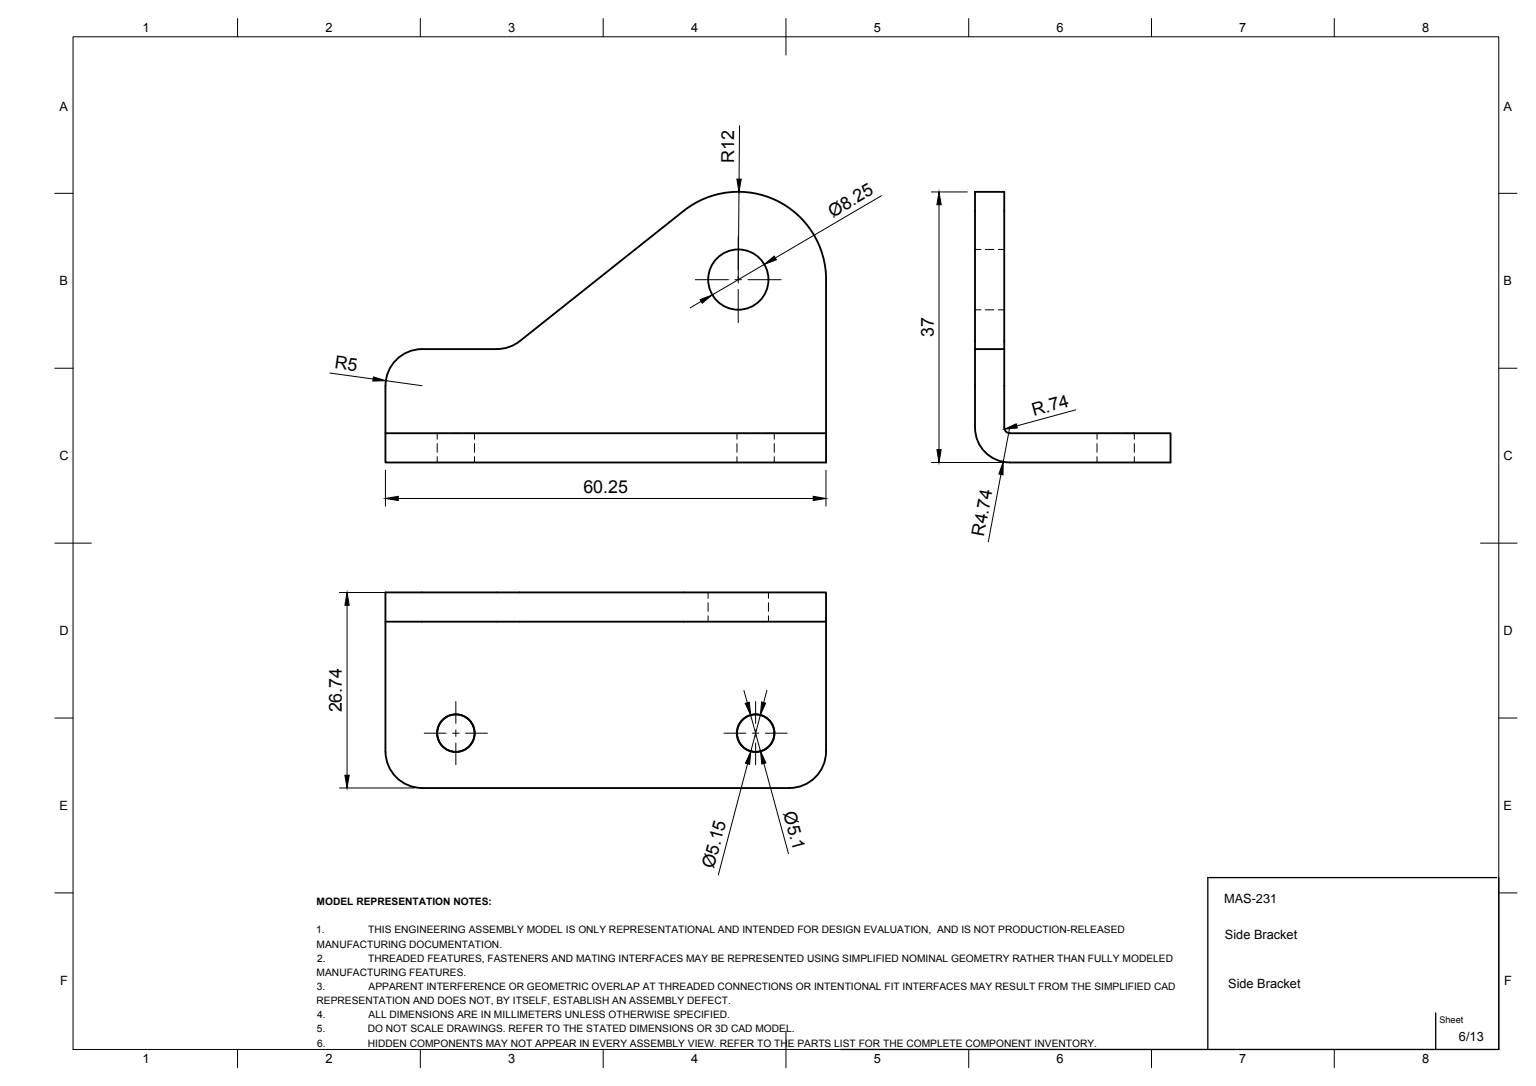
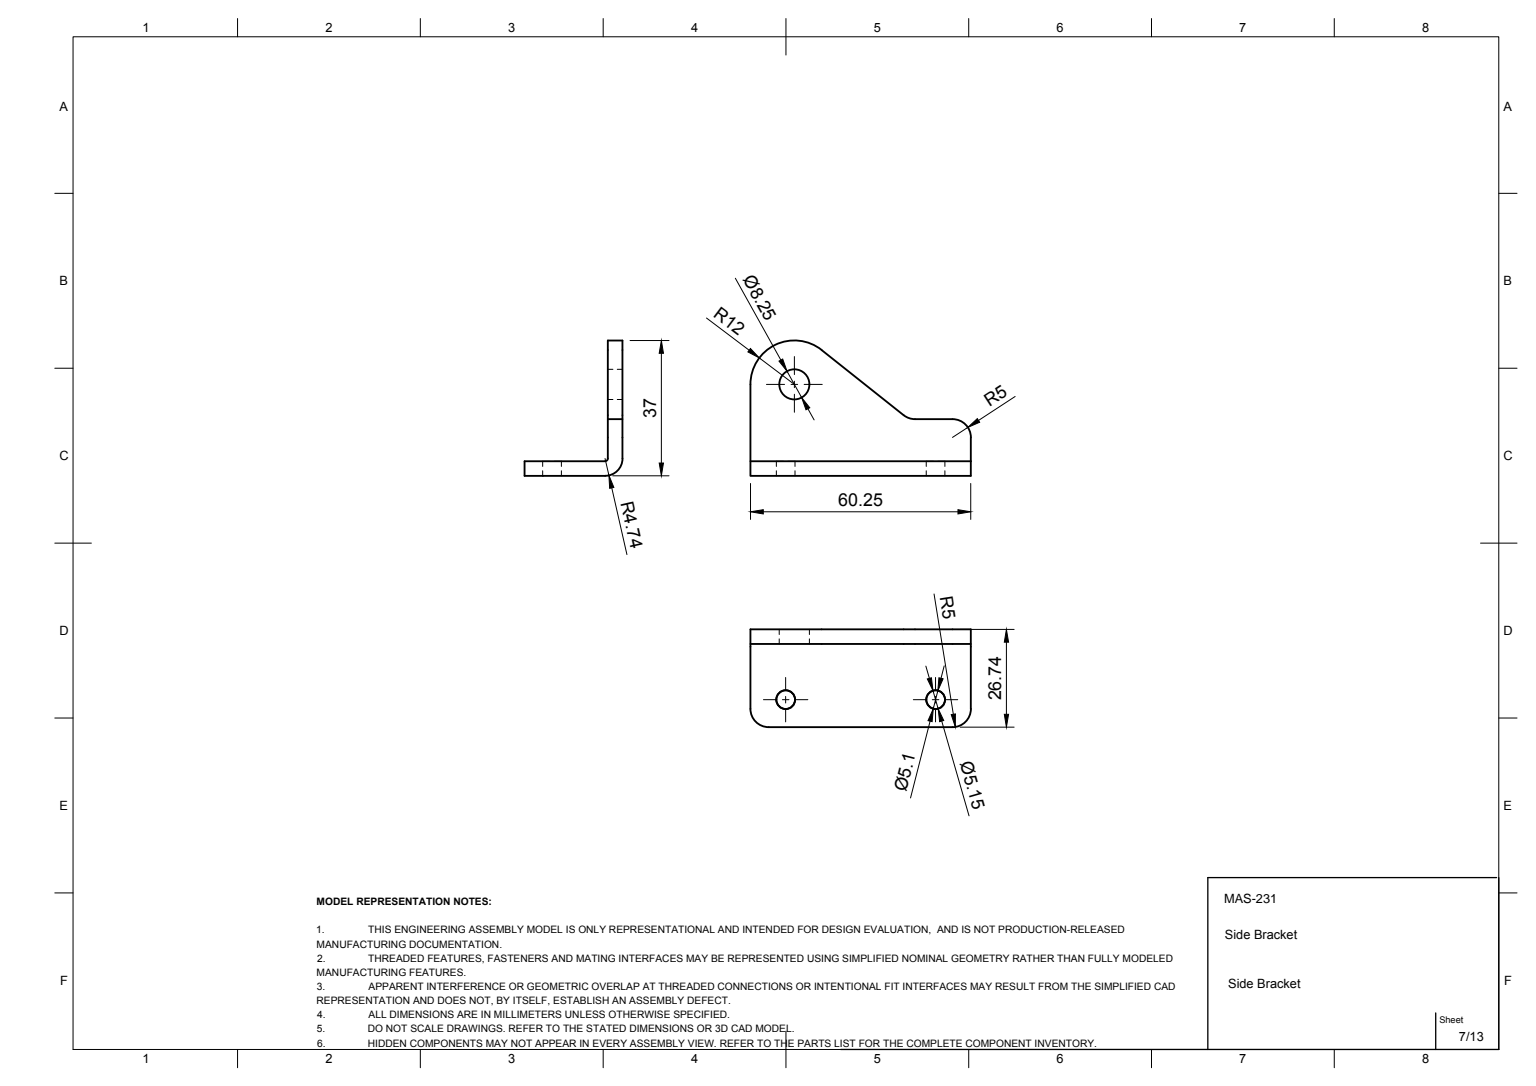
ISO-10303-21;
HEADER;
FILE_DESCRIPTION (('STEP AP214'),
    '1' );
FILE_NAME ( 'Side Bracket.step', '2026-10-04T02:08:54', ( '' ), ( '' ), 'STEP AP214', 'Unspecified', '' );
FILE_SCHEMA (( 'AUTOMOTIVE_DESIGN' ));
ENDSEC;
DATA;
#26=DIRECTION ( 'NONE',  ( 0.000000000000000000, 0.000000000000000000, -1.000000000000000000 ) ) ;
#60=VECTOR ( 'NONE', #5427, 39.37007874015748143 ) ;
#113=CARTESIAN_POINT ( 'NONE',  ( -0.6195511811023656223, 0.6102362204724407491, 1.186023622047243986 ) ) ;
#127=ORIENTED_EDGE ( 'NONE', *, *, #14895, .F. ) ;
#130=ADVANCED_FACE ( 'NONE', ( #15231 ), #18799, .T. ) ;
#143=DIRECTION ( 'NONE',  ( -0.000000000000000000, -0.000000000000000000, 1.000000000000000000 ) ) ;
#260=VECTOR ( 'NONE', #32837, 39.37007874015748143 ) ;
#351=DIRECTION ( 'NONE',  ( 0.000000000000000000, -0.6220299971367094782, 0.7829934116339071215 ) ) ;
#414=CARTESIAN_POINT ( 'NONE',  ( -0.4330708661417322913, 0.1574803149606299191, 1.186023622047243986 ) ) ;
#512=CARTESIAN_POINT ( 'NONE',  ( 0.1377952755905511861, -1.365923996832131609E-16, 0.9074803149606294195 ) ) ;
#523=ADVANCED_FACE ( 'NONE', ( #24362 ), #19359, .F. ) ;
#529=VERTEX_POINT ( 'NONE', #25560 ) ;
#593=CARTESIAN_POINT ( 'NONE',  ( -0.4620708661417322616, 0.6102362204724408601, 0.5854071585544579071 ) ) ;
#637=CARTESIAN_POINT ( 'NONE',  ( 0.1377952755905511861, 0.1574803149606299191, -0.7057086614173228023 ) ) ;
#705=DIRECTION ( 'NONE',  ( 0.000000000000000000, -1.000000000000000000, 0.000000000000000000 ) ) ;
#817=CIRCLE ( 'NONE', #6954, 0.1624015748031501782 ) ;
#870=DIRECTION ( 'NONE',  ( 1.000000000000000000, 0.000000000000000000, 0.000000000000000000 ) ) ;
#892=ORIENTED_EDGE ( 'NONE', *, *, #28438, .F. ) ;
#899=EDGE_CURVE ( 'NONE', #2549, #11279, #11446, .T. ) ;
#1038=CARTESIAN_POINT ( 'NONE',  ( 0.2362204724409448509, 0.000000000000000000, 0.9891732283464566011 ) ) ;
#1123=EDGE_CURVE ( 'NONE', #29994, #13605, #35169, .T. ) ;
#1148=VECTOR ( 'NONE', #44501, 39.37007874015748143 ) ;
#1243=AXIS2_PLACEMENT_3D ( 'NONE', #9459, #1527, #38204 ) ;
#1300=EDGE_CURVE ( 'NONE', #29883, #25085, #16051, .T. ) ;
#1356=ADVANCED_FACE ( 'NONE', ( #19336 ), #22697, .T. ) ;
#1362=LINE ( 'NONE', #9042, #21868 ) ;
#1430=DIRECTION ( 'NONE',  ( -0.000000000000000000, 1.000000000000000000, -0.000000000000000000 ) ) ;
#1435=AXIS2_PLACEMENT_3D ( 'NONE', #9624, #2406, #9388 ) ;
#1436=FACE_OUTER_BOUND ( 'NONE', #45627, .T. ) ;
#1527=DIRECTION ( 'NONE',  ( -1.000000000000000000, 0.000000000000000000, 0.000000000000000000 ) ) ;
#1544=CARTESIAN_POINT ( 'NONE',  ( -0.6195511811023656223, 1.354170115732555191, -0.4197102375732078561 ) ) ;
#1632=DIRECTION ( 'NONE',  ( 1.000000000000000000, 0.000000000000000000, 0.000000000000000000 ) ) ;
#1732=CARTESIAN_POINT ( 'NONE',  ( 0.2362204724409448509, 0.1574803149606299191, -1.186023622047243986 ) ) ;
#1811=CARTESIAN_POINT ( 'NONE',  ( -0.6195511811023656223, 0.6102362204724407491, 0.9891732283464566011 ) ) ;
#1826=FACE_OUTER_BOUND ( 'NONE', #11922, .T. ) ;
#1835=EDGE_LOOP ( 'NONE', ( #32627, #33041, #45588, #11414 ) ) ;
#1873=EDGE_CURVE ( 'NONE', #12155, #6854, #31803, .T. ) ;
#1938=VECTOR ( 'NONE', #4599, 39.37007874015748143 ) ;
#1969=DIRECTION ( 'NONE',  ( 0.000000000000000000, 0.000000000000000000, -1.000000000000000000 ) ) ;
#2028=DIRECTION ( 'NONE',  ( -1.000000000000000000, 0.000000000000000000, -0.000000000000000000 ) ) ;
#2073=ORIENTED_EDGE ( 'NONE', *, *, #24705, .F. ) ;
#2106=CARTESIAN_POINT ( 'NONE',  ( 0.1377952755905511861, 0.1574803149606299191, -0.8070866141732283561 ) ) ;
#2154=CYLINDRICAL_SURFACE ( 'NONE', #8738, 0.1003937007874010356 ) ;
#2261=ORIENTED_EDGE ( 'NONE', *, *, #17908, .T. ) ;
#2280=DIRECTION ( 'NONE',  ( 1.000000000000000000, 0.000000000000000000, 0.000000000000000000 ) ) ;
#2397=DIRECTION ( 'NONE',  ( 0.000000000000000000, -1.000000000000000000, 0.000000000000000000 ) ) ;
#2406=DIRECTION ( 'NONE',  ( 1.000000000000000000, 0.000000000000000000, 0.000000000000000000 ) ) ;
#2549=VERTEX_POINT ( 'NONE', #15817 ) ;
#2607=DIRECTION ( 'NONE',  ( 0.000000000000000000, 0.7071067811862592478, 0.7071067811868357866 ) ) ;
#2639=ADVANCED_FACE ( 'NONE', ( #36141 ), #42143, .F. ) ;
#2693=FACE_OUTER_BOUND ( 'NONE', #5912, .T. ) ;
#2716=CARTESIAN_POINT ( 'NONE',  ( 0.1377952755905511861, 0.1574803149606299191, 0.8070866141732283561 ) ) ;
#2735=AXIS2_PLACEMENT_3D ( 'NONE', #15622, #15860, #22308 ) ;
#2768=EDGE_LOOP ( 'NONE', ( #37512, #34957, #12199, #30879 ) ) ;
#2804=CARTESIAN_POINT ( 'NONE',  ( -0.6195511811023656223, 0.4133858267716533086, 0.9891732283464566011 ) ) ;
#2834=EDGE_LOOP ( 'NONE', ( #20225, #46223, #10055, #19298 ) ) ;
#2905=EDGE_CURVE ( 'NONE', #13605, #29883, #29414, .T. ) ;
#2998=DIRECTION ( 'NONE',  ( 1.000000000000000000, 0.000000000000000000, 0.000000000000000000 ) ) ;
#3054=DIRECTION ( 'NONE',  ( -0.000000000000000000, 1.000000000000000000, -0.000000000000000000 ) ) ;
#3076=EDGE_CURVE ( 'NONE', #35796, #18058, #15219, .T. ) ;
#3124=DIRECTION ( 'NONE',  ( -1.000000000000000000, -0.000000000000000000, -0.000000000000000000 ) ) ;
#3183=EDGE_CURVE ( 'NONE', #44249, #11279, #817, .T. ) ;
#3184=LINE ( 'NONE', #15175, #34310 ) ;
#3567=CARTESIAN_POINT ( 'NONE',  ( -0.4330708661417322913, 0.1574803149606299191, -1.186023622047243986 ) ) ;
#3624=ORIENTED_EDGE ( 'NONE', *, *, #6205, .F. ) ;
#3645=DIRECTION ( 'NONE',  ( 1.000000000000000000, -0.000000000000000000, -0.000000000000000000 ) ) ;
#3647=CARTESIAN_POINT ( 'NONE',  ( 0.1377952755905511861, 0.1574803149606299191, 0.8070866141732283561 ) ) ;
#3695=CARTESIAN_POINT ( 'NONE',  ( 0.2362204724409448509, 0.000000000000000000, -0.9891732283464566011 ) ) ;
#3759=DIRECTION ( 'NONE',  ( 0.000000000000000000, 0.000000000000000000, -1.000000000000000000 ) ) ;
#3854=ORIENTED_EDGE ( 'NONE', *, *, #16088, .T. ) ;
#3953=VERTEX_POINT ( 'NONE', #21496 ) ;
#4011=LINE ( 'NONE', #414, #45904 ) ;
#4021=AXIS2_PLACEMENT_3D ( 'NONE', #30055, #45315, #26672 ) ;
#4101=CARTESIAN_POINT ( 'NONE',  ( -0.6195511811023656223, 0.9842519685039375910, -0.7135826771653542844 ) ) ;
#4124=VERTEX_POINT ( 'NONE', #31468 ) ;
#4374=LINE ( 'NONE', #44870, #28589 ) ;
#4399=DIRECTION ( 'NONE',  ( 0.000000000000000000, -6.938893903907227392E-16, -1.000000000000000000 ) ) ;
#4455=AXIS2_PLACEMENT_3D ( 'NONE', #5889, #2280, #16908 ) ;
#4484=FACE_BOUND ( 'NONE', #14477, .T. ) ;
#4496=LINE ( 'NONE', #22739, #29482 ) ;
#4526=ADVANCED_FACE ( 'NONE', ( #12501 ), #2154, .F. ) ;
#4599=DIRECTION ( 'NONE',  ( 0.000000000000000000, 0.000000000000000000, -1.000000000000000000 ) ) ;
#4652=DIRECTION ( 'NONE',  ( 1.000000000000000000, -0.000000000000000000, -0.000000000000000000 ) ) ;
#4705=CARTESIAN_POINT ( 'NONE',  ( 0.1377952755905511861, 0.1564960629921262614, 0.8070866141732283561 ) ) ;
#4711=DIRECTION ( 'NONE',  ( 0.000000000000000000, -1.000000000000000000, 0.000000000000000000 ) ) ;
#4718=DIRECTION ( 'NONE',  ( -0.000000000000000000, 0.000000000000000000, 1.000000000000000000 ) ) ;
#4878=LINE ( 'NONE', #19504, #35583 ) ;
#4897=UNCERTAINTY_MEASURE_WITH_UNIT (LENGTH_MEASURE( 1.000000000000000082E-05 ), #37648, 'distance_accuracy_value', 'NONE') ;
#5034=AXIS2_PLACEMENT_3D ( 'NONE', #41786, #27710, #8985 ) ;
#5051=( LENGTH_UNIT ( ) NAMED_UNIT ( * ) SI_UNIT ( $, .METRE. ) ) ;
#5079=VERTEX_POINT ( 'NONE', #20073 ) ;
#5202=AXIS2_PLACEMENT_3D ( 'NONE', #8256, #4652, #37974 ) ;
#5208=CARTESIAN_POINT ( 'NONE',  ( 0.1377952755905512139, -1.365923996832131609E-16, -0.9074803149606294195 ) ) ;
#5223=CARTESIAN_POINT ( 'NONE',  ( -0.6195511811023656223, 0.000000000000000000, -1.186023622047243986 ) ) ;
#5224=CARTESIAN_POINT ( 'NONE',  ( -0.6195511811023656223, 0.4133858267716533086, 0.9891732283464566011 ) ) ;
#5284=PRESENTATION_STYLE_ASSIGNMENT (( #30489 ) ) ;
#5294=AXIS2_PLACEMENT_3D ( 'NONE', #3647, #25483, #21871 ) ;
#5427=DIRECTION ( 'NONE',  ( 1.000000000000000000, -0.000000000000000000, -0.000000000000000000 ) ) ;
#5572=CIRCLE ( 'NONE', #4021, 0.1624015748031501782 ) ;
#5598=DIRECTION ( 'NONE',  ( 0.000000000000000000, 0.000000000000000000, -1.000000000000000000 ) ) ;
#5659=CARTESIAN_POINT ( 'NONE',  ( 0.2362204724409448509, 0.1574803149606299191, -0.9891732283464566011 ) ) ;
#5702=CARTESIAN_POINT ( 'NONE',  ( 0.2362204724409448509, 0.000000000000000000, -0.9891732283464566011 ) ) ;
#5731=ORIENTED_EDGE ( 'NONE', *, *, #10353, .F. ) ;
#5743=DIRECTION ( 'NONE',  ( 8.659560562358463011E-17, 0.7071067811862592478, -0.7071067811868357866 ) ) ;
#5889=CARTESIAN_POINT ( 'NONE',  ( -0.6195511811023656223, 0.9842519685039370358, -0.7135826771653542844 ) ) ;
#5896=DIRECTION ( 'NONE',  ( -0.000000000000000000, 1.000000000000000000, -0.000000000000000000 ) ) ;
#5907=DIRECTION ( 'NONE',  ( 0.000000000000000000, 0.000000000000000000, 1.000000000000000000 ) ) ;
#5912=EDGE_LOOP ( 'NONE', ( #30515, #10422, #17857, #42784, #24375, #36154, #43440, #45182 ) ) ;
#5941=ORIENTED_EDGE ( 'NONE', *, *, #12634, .F. ) ;
#6011=EDGE_CURVE ( 'NONE', #43147, #15333, #1362, .T. ) ;
#6110=LINE ( 'NONE', #20734, #24316 ) ;
#6132=APPLICATION_CONTEXT ( 'automotive_design' ) ;
#6153=ORIENTED_EDGE ( 'NONE', *, *, #39860, .F. ) ;
#6205=EDGE_CURVE ( 'NONE', #22637, #43357, #7336, .T. ) ;
#6242=VECTOR ( 'NONE', #22207, 39.37007874015748143 ) ;
#6259=EDGE_CURVE ( 'NONE', #11279, #44249, #37154, .T. ) ;
#6289=DIRECTION ( 'NONE',  ( 0.000000000000000000, 1.000000000000000000, 0.000000000000000000 ) ) ;
#6308=LINE ( 'NONE', #24538, #22934 ) ;
#6350=ORIENTED_EDGE ( 'NONE', *, *, #35400, .T. ) ;
#6362=FACE_OUTER_BOUND ( 'NONE', #32085, .T. ) ;
#6381=EDGE_CURVE ( 'NONE', #3953, #17273, #33360, .T. ) ;
#6389=AXIS2_PLACEMENT_3D ( 'NONE', #21796, #15565, #30204 ) ;
#6414=CARTESIAN_POINT ( 'NONE',  ( 0.1377952755905512139, 0.1574803149606299191, 0.7066929133858274037 ) ) ;
#6442=ADVANCED_FACE ( 'NONE', ( #8507 ), #24088, .T. ) ;
#6446=EDGE_LOOP ( 'NONE', ( #33560, #24619, #11277, #8369 ) ) ;
#6451=DIRECTION ( 'NONE',  ( 0.000000000000000000, -0.000000000000000000, -1.000000000000000000 ) ) ;
#6518=CIRCLE ( 'NONE', #8063, 0.1013779527559055538 ) ;
#6533=DIRECTION ( 'NONE',  ( 0.000000000000000000, 1.000000000000000000, 0.000000000000000000 ) ) ;
#6658=FACE_OUTER_BOUND ( 'NONE', #42482, .T. ) ;
#6854=VERTEX_POINT ( 'NONE', #17889 ) ;
#6882=EDGE_LOOP ( 'NONE', ( #7362, #23755 ) ) ;
#6954=AXIS2_PLACEMENT_3D ( 'NONE', #43531, #25355, #3759 ) ;
#6982=CARTESIAN_POINT ( 'NONE',  ( 0.4330708661417322913, 0.1574803149606299191, -0.9891732283464566011 ) ) ;
#7140=CARTESIAN_POINT ( 'NONE',  ( 0.4330708661417322913, 0.000000000000000000, 0.9891732283464566011 ) ) ;
#7228=LENGTH_MEASURE_WITH_UNIT ( LENGTH_MEASURE( 0.02539999999999999897 ), #7455 ) ;
#7255=CARTESIAN_POINT ( 'NONE',  ( 0.2362204724409448509, 0.1574803149606299191, 1.186023622047243986 ) ) ;
#7294=FACE_OUTER_BOUND ( 'NONE', #24349, .T. ) ;
#7336=CIRCLE ( 'NONE', #16503, 0.1968503937007874405 ) ;
#7362=ORIENTED_EDGE ( 'NONE', *, *, #29891, .T. ) ;
#7455=( LENGTH_UNIT ( ) NAMED_UNIT ( * ) SI_UNIT ( $, .METRE. ) ) ;
#7562=DIRECTION ( 'NONE',  ( -1.000000000000000000, 0.000000000000000000, 0.000000000000000000 ) ) ;
#7622=EDGE_CURVE ( 'NONE', #42395, #24436, #30308, .T. ) ;
#7641=DIRECTION ( 'NONE',  ( 0.000000000000000000, 0.000000000000000000, 1.000000000000000000 ) ) ;
#7694=AXIS2_PLACEMENT_3D ( 'NONE', #31721, #9673, #17552 ) ;
#7700=CARTESIAN_POINT ( 'NONE',  ( 0.1377952755905511861, -1.365923996832131609E-16, 0.8070866141732283561 ) ) ;
#7771=DIRECTION ( 'NONE',  ( -1.000000000000000000, -0.000000000000000000, -0.000000000000000000 ) ) ;
#7800=CARTESIAN_POINT ( 'NONE',  ( 0.2362204724409448509, 0.1574803149606299191, 0.9891732283464566011 ) ) ;
#7922=ORIENTED_EDGE ( 'NONE', *, *, #14949, .F. ) ;
#8001=CARTESIAN_POINT ( 'NONE',  ( 0.1377952755905511861, 0.1564960629921262614, -0.8070866141732283561 ) ) ;
#8030=DIRECTION ( 'NONE',  ( 1.000000000000000000, -0.000000000000000000, -0.000000000000000000 ) ) ;
#8063=AXIS2_PLACEMENT_3D ( 'NONE', #8148, #705, #15363 ) ;
#8148=CARTESIAN_POINT ( 'NONE',  ( 0.1377952755905511861, 0.1574803149606299191, -0.8070866141732283561 ) ) ;
#8167=DIRECTION ( 'NONE',  ( 0.000000000000000000, 0.000000000000000000, 1.000000000000000000 ) ) ;
#8193=ORIENTED_EDGE ( 'NONE', *, *, #31586, .T. ) ;
#8253=DIRECTION ( 'NONE',  ( -0.000000000000000000, 0.7829934116339072325, 0.6220299971367095893 ) ) ;
#8256=CARTESIAN_POINT ( 'NONE',  ( -0.4620708661417322616, 0.9842519685039375910, -0.7135826771653542844 ) ) ;
#8369=ORIENTED_EDGE ( 'NONE', *, *, #27138, .F. ) ;
#8417=ORIENTED_EDGE ( 'NONE', *, *, #28893, .F. ) ;
#8475=CIRCLE ( 'NONE', #33010, 0.1864803149606299171 ) ;
#8507=FACE_OUTER_BOUND ( 'NONE', #29134, .T. ) ;
#8581=CIRCLE ( 'NONE', #24674, 0.1624015748031501782 ) ;
#8585=CARTESIAN_POINT ( 'NONE',  ( -0.4330708661417356775, 0.1864803149606299171, 1.186023622047243986 ) ) ;
#8653=EDGE_CURVE ( 'NONE', #43692, #16170, #6518, .T. ) ;
#8709=ORIENTED_EDGE ( 'NONE', *, *, #11424, .F. ) ;
#8738=AXIS2_PLACEMENT_3D ( 'NONE', #44808, #1430, #41675 ) ;
#8756=EDGE_CURVE ( 'NONE', #35268, #16170, #24432, .T. ) ;
#8833=LINE ( 'NONE', #5223, #25116 ) ;
#8834=FACE_OUTER_BOUND ( 'NONE', #6446, .T. ) ;
#8855=ORIENTED_EDGE ( 'NONE', *, *, #40556, .F. ) ;
#8985=DIRECTION ( 'NONE',  ( 0.000000000000000000, 0.000000000000000000, 1.000000000000000000 ) ) ;
#9042=CARTESIAN_POINT ( 'NONE',  ( 0.1377952755905512139, 0.1574803149606299191, -0.9074803149606294195 ) ) ;
#9307=EDGE_CURVE ( 'NONE', #12155, #29873, #41016, .T. ) ;
#9322=ORIENTED_EDGE ( 'NONE', *, *, #2905, .F. ) ;
#9377=FACE_BOUND ( 'NONE', #18186, .T. ) ;
#9388=DIRECTION ( 'NONE',  ( 0.000000000000000000, 0.000000000000000000, -1.000000000000000000 ) ) ;
#9459=CARTESIAN_POINT ( 'NONE',  ( 0.4330708661417322913, 0.000000000000000000, 0.000000000000000000 ) ) ;
#9573=CARTESIAN_POINT ( 'NONE',  ( -0.4620708661417322616, 0.6529540528279709211, 0.4629603087243971959 ) ) ;
#9624=CARTESIAN_POINT ( 'NONE',  ( -0.6195511811023656223, 0.8070866141732282451, 0.5854071585544579071 ) ) ;
#9633=ORIENTED_EDGE ( 'NONE', *, *, #47238, .F. ) ;
#9643=ORIENTED_EDGE ( 'NONE', *, *, #26702, .F. ) ;
#9673=DIRECTION ( 'NONE',  ( 1.000000000000000000, 0.000000000000000000, 0.000000000000000000 ) ) ;
#9681=DIRECTION ( 'NONE',  ( 1.000000000000000000, 0.000000000000000000, 0.000000000000000000 ) ) ;
#9700=ORIENTED_EDGE ( 'NONE', *, *, #20244, .T. ) ;
#9746=DIRECTION ( 'NONE',  ( 1.000000000000000000, 0.000000000000000000, 0.000000000000000000 ) ) ;
#9869=EDGE_LOOP ( 'NONE', ( #5731, #22652, #45000, #25793 ) ) ;
#9905=LINE ( 'NONE', #39113, #37079 ) ;
#9974=DIRECTION ( 'NONE',  ( 0.000000000000000000, 0.000000000000000000, -1.000000000000000000 ) ) ;
#9992=ORIENTED_EDGE ( 'NONE', *, *, #14895, .T. ) ;
#10018=DIRECTION ( 'NONE',  ( 0.000000000000000000, 0.000000000000000000, -1.000000000000000000 ) ) ;
#10032=AXIS2_PLACEMENT_3D ( 'NONE', #5224, #19854, #27798 ) ;
#10055=ORIENTED_EDGE ( 'NONE', *, *, #3183, .T. ) ;
#10270=DIRECTION ( 'NONE',  ( -0.000000000000000000, 1.000000000000000000, -0.000000000000000000 ) ) ;
#10274=LINE ( 'NONE', #7140, #25258 ) ;
#10313=DIRECTION ( 'NONE',  ( 0.000000000000000000, 0.000000000000000000, -1.000000000000000000 ) ) ;
#10353=EDGE_CURVE ( 'NONE', #3953, #40227, #17444, .T. ) ;
#10422=ORIENTED_EDGE ( 'NONE', *, *, #22465, .T. ) ;
#10470=ORIENTED_EDGE ( 'NONE', *, *, #20770, .T. ) ;
#10479=ORIENTED_EDGE ( 'NONE', *, *, #6205, .T. ) ;
#10502=CARTESIAN_POINT ( 'NONE',  ( -0.6195511811023656223, 0.1864803149606299171, -1.186023622047243986 ) ) ;
#10505=DIRECTION ( 'NONE',  ( -1.000000000000000000, -0.000000000000000000, -0.000000000000000000 ) ) ;
#10513=CYLINDRICAL_SURFACE ( 'NONE', #36435, 0.1003937007874010356 ) ;
#10628=EDGE_CURVE ( 'NONE', #13680, #25085, #6110, .T. ) ;
#10784=ORIENTED_EDGE ( 'NONE', *, *, #6381, .T. ) ;
#10835=DIRECTION ( 'NONE',  ( 1.000000000000000000, 0.000000000000000000, 0.000000000000000000 ) ) ;
#10911=DIRECTION ( 'NONE',  ( 0.000000000000000000, 0.000000000000000000, -1.000000000000000000 ) ) ;
#11221=ADVANCED_FACE ( 'NONE', ( #41058 ), #19033, .F. ) ;
#11265=FACE_BOUND ( 'NONE', #46562, .T. ) ;
#11277=ORIENTED_EDGE ( 'NONE', *, *, #22465, .F. ) ;
#11279=VERTEX_POINT ( 'NONE', #20461 ) ;
#11414=ORIENTED_EDGE ( 'NONE', *, *, #6259, .T. ) ;
#11424=EDGE_CURVE ( 'NONE', #25085, #29994, #3184, .T. ) ;
#11446=LINE ( 'NONE', #37295, #19059 ) ;
#11453=DIRECTION ( 'NONE',  ( 0.000000000000000000, 0.000000000000000000, -1.000000000000000000 ) ) ;
#11510=ORIENTED_EDGE ( 'NONE', *, *, #25210, .F. ) ;
#11597=DIRECTION ( 'NONE',  ( 0.000000000000000000, 0.7071067811862592478, 0.7071067811868357866 ) ) ;
#11712=DIRECTION ( 'NONE',  ( 1.000000000000000000, 0.000000000000000000, 0.000000000000000000 ) ) ;
#11733=CARTESIAN_POINT ( 'NONE',  ( -0.4620708661417322616, 0.9842519685039375910, -0.7135826771653542844 ) ) ;
#11743=ORIENTED_EDGE ( 'NONE', *, *, #20979, .F. ) ;
#11787=( NAMED_UNIT ( * ) SI_UNIT ( $, .STERADIAN. ) SOLID_ANGLE_UNIT ( ) ) ;
#11794=( NAMED_UNIT ( * ) PLANE_ANGLE_UNIT ( ) SI_UNIT ( $, .RADIAN. ) ) ;
#11827=EDGE_LOOP ( 'NONE', ( #32231, #43129, #27996, #7922 ) ) ;
#11859=CARTESIAN_POINT ( 'NONE',  ( -0.6195511811023656223, 0.6102362204724408601, 0.5854071585544579071 ) ) ;
#11877=ORIENTED_EDGE ( 'NONE', *, *, #17908, .F. ) ;
#11922=EDGE_LOOP ( 'NONE', ( #18416, #10479, #15708, #9700, #46879, #16747 ) ) ;
#11944=PRODUCT_DEFINITION ( 'UNKNOWN', '', #26300, #18289 ) ;
#12098=CIRCLE ( 'NONE', #24332, 0.1003937007874010356 ) ;
#12155=VERTEX_POINT ( 'NONE', #16762 ) ;
#12190=CIRCLE ( 'NONE', #39696, 0.1968503937007874405 ) ;
#12199=ORIENTED_EDGE ( 'NONE', *, *, #45641, .F. ) ;
#12200=CYLINDRICAL_SURFACE ( 'NONE', #33811, 0.1864803149606299171 ) ;
#12253=VERTEX_POINT ( 'NONE', #38327 ) ;
#12448=CIRCLE ( 'NONE', #32360, 0.1864803149606299448 ) ;
#12501=FACE_OUTER_BOUND ( 'NONE', #9869, .T. ) ;
#12510=SURFACE_SIDE_STYLE ('',( #34082 ) ) ;
#12551=DIRECTION ( 'NONE',  ( -1.000000000000000000, 0.000000000000000000, 0.000000000000000000 ) ) ;
#12558=CARTESIAN_POINT ( 'NONE',  ( 0.1377952755905512139, 0.1574803149606299191, -0.9084645669291339098 ) ) ;
#12600=EDGE_LOOP ( 'NONE', ( #35339, #13655, #8417, #36103 ) ) ;
#12634=EDGE_CURVE ( 'NONE', #15333, #43692, #15848, .T. ) ;
#12815=CARTESIAN_POINT ( 'NONE',  ( 0.1377952755905511861, 0.1564960629921262614, 0.8070866141732283561 ) ) ;
#12911=DIRECTION ( 'NONE',  ( 0.000000000000000000, 1.000000000000000000, 0.000000000000000000 ) ) ;
#12994=CARTESIAN_POINT ( 'NONE',  ( 0.4330708661417322913, 0.1574803149606299191, 1.186023622047243986 ) ) ;
#13111=CARTESIAN_POINT ( 'NONE',  ( 0.4330708661417322913, 0.000000000000000000, 0.9891732283464564901 ) ) ;
#13161=DIRECTION ( 'NONE',  ( 0.000000000000000000, 0.000000000000000000, -1.000000000000000000 ) ) ;
#13215=COLOUR_RGB ( '', 0.66274510, 0.83137255, 0.94901961) ;
#13306=ORIENTED_EDGE ( 'NONE', *, *, #44495, .F. ) ;
#13461=CARTESIAN_POINT ( 'NONE',  ( 0.1377952755905512139, 0.1564960629921262614, -0.9074803149606294195 ) ) ;
#13564=CARTESIAN_POINT ( 'NONE',  ( -0.6195511811023656223, 0.000000000000000000, 1.186023622047243986 ) ) ;
#13605=VERTEX_POINT ( 'NONE', #593 ) ;
#13645=ADVANCED_FACE ( 'NONE', ( #17881 ), #29200, .F. ) ;
#13655=ORIENTED_EDGE ( 'NONE', *, *, #33256, .T. ) ;
#13680=VERTEX_POINT ( 'NONE', #1544 ) ;
#13729=CARTESIAN_POINT ( 'NONE',  ( -0.4620708661417322616, 0.9842519685039370358, -1.186023622047243986 ) ) ;
#13748=ORIENTED_EDGE ( 'NONE', *, *, #33855, .F. ) ;
#13760=ORIENTED_EDGE ( 'NONE', *, *, #24727, .F. ) ;
#13795=EDGE_LOOP ( 'NONE', ( #27097, #46225, #17036, #10470 ) ) ;
#13889=CARTESIAN_POINT ( 'NONE',  ( -0.4620708661417322616, 0.1864803149606299448, -0.7135826771653542844 ) ) ;
#13892=AXIS2_PLACEMENT_3D ( 'NONE', #21219, #21709, #43737 ) ;
#13933=ORIENTED_EDGE ( 'NONE', *, *, #16088, .F. ) ;
#13934=AXIS2_PLACEMENT_3D ( 'NONE', #2804, #10505, #10018 ) ;
#13957=DIRECTION ( 'NONE',  ( 8.659560562358463011E-17, 0.7071067811862592478, -0.7071067811868357866 ) ) ;
#14001=FACE_OUTER_BOUND ( 'NONE', #19415, .T. ) ;
#14164=ORIENTED_EDGE ( 'NONE', *, *, #30136, .F. ) ;
#14214=PLANE ( 'NONE',  #7694 ) ;
#14338=CARTESIAN_POINT ( 'NONE',  ( 0.1377952755905511861, 0.1564960629921262614, 0.8070866141732283561 ) ) ;
#14343=CYLINDRICAL_SURFACE ( 'NONE', #40544, 0.1003937007874010356 ) ;
#14419=AXIS2_PLACEMENT_3D ( 'NONE', #29743, #40457, #7641 ) ;
#14477=EDGE_LOOP ( 'NONE', ( #29063, #6350 ) ) ;
#14589=CARTESIAN_POINT ( 'NONE',  ( 0.4330708661417322913, 0.000000000000000000, -0.9891732283464566011 ) ) ;
#14590=PRODUCT ( 'Side Bracket', 'Side Bracket', '', ( #16610 ) ) ;
#14602=PLANE ( 'NONE',  #6389 ) ;
#14607=CARTESIAN_POINT ( 'NONE',  ( -0.4620708661417322616, 0.1864803149606299448, 1.186023622047243986 ) ) ;
#14748=CARTESIAN_POINT ( 'NONE',  ( -0.4620708661417322616, 0.8070866141732282451, 0.5854071585544579071 ) ) ;
#14752=DIRECTION ( 'NONE',  ( 1.000000000000000000, 0.000000000000000000, 0.000000000000000000 ) ) ;
#14895=EDGE_CURVE ( 'NONE', #46399, #37690, #6308, .T. ) ;
#14949=EDGE_CURVE ( 'NONE', #46224, #24436, #18354, .T. ) ;
#15079=VERTEX_POINT ( 'NONE', #30062 ) ;
#15167=ORIENTED_EDGE ( 'NONE', *, *, #46577, .T. ) ;
#15175=CARTESIAN_POINT ( 'NONE',  ( -0.4620708661417322616, 0.6529540528279709211, 0.4629603087243968074 ) ) ;
#15219=LINE ( 'NONE', #29868, #42913 ) ;
#15231=FACE_OUTER_BOUND ( 'NONE', #2768, .T. ) ;
#15258=AXIS2_PLACEMENT_3D ( 'NONE', #44021, #870, #11453 ) ;
#15298=CARTESIAN_POINT ( 'NONE',  ( -0.4330708661417322913, 0.1864803149606299448, 1.186023622047243986 ) ) ;
#15333=VERTEX_POINT ( 'NONE', #13461 ) ;
#15363=DIRECTION ( 'NONE',  ( 0.000000000000000000, 0.000000000000000000, -1.000000000000000000 ) ) ;
#15565=DIRECTION ( 'NONE',  ( 1.000000000000000000, 0.000000000000000000, 0.000000000000000000 ) ) ;
#15622=CARTESIAN_POINT ( 'NONE',  ( 0.1377952755905511861, 0.1574803149606299191, 0.8070866141732283561 ) ) ;
#15675=CARTESIAN_POINT ( 'NONE',  ( -0.4330708661417322913, 0.1574803149606299191, 1.186023622047243986 ) ) ;
#15696=DIRECTION ( 'NONE',  ( 0.000000000000000000, -1.000000000000000000, 0.000000000000000000 ) ) ;
#15705=ORIENTED_EDGE ( 'NONE', *, *, #1123, .F. ) ;
#15708=ORIENTED_EDGE ( 'NONE', *, *, #18654, .F. ) ;
#15817=CARTESIAN_POINT ( 'NONE',  ( -0.6195511811023656223, 0.9842519685039375910, -0.8759842519685044904 ) ) ;
#15848=LINE ( 'NONE', #38575, #38153 ) ;
#15860=DIRECTION ( 'NONE',  ( -0.000000000000000000, 1.000000000000000000, -0.000000000000000000 ) ) ;
#16016=DIRECTION ( 'NONE',  ( -0.000000000000000000, 1.000000000000000000, -0.000000000000000000 ) ) ;
#16051=CIRCLE ( 'NONE', #1435, 0.1968503937007874405 ) ;
#16088=EDGE_CURVE ( 'NONE', #6854, #22637, #43559, .T. ) ;
#16170=VERTEX_POINT ( 'NONE', #637 ) ;
#16189=VECTOR ( 'NONE', #7771, 39.37007874015748143 ) ;
#16233=ORIENTED_EDGE ( 'NONE', *, *, #18654, .T. ) ;
#16315=EDGE_CURVE ( 'NONE', #44357, #42566, #4011, .T. ) ;
#16429=CARTESIAN_POINT ( 'NONE',  ( -0.6195511811023656223, 0.000000000000000000, -1.186023622047243986 ) ) ;
#16468=PLANE ( 'NONE',  #26881 ) ;
#16503=AXIS2_PLACEMENT_3D ( 'NONE', #7800, #19292, #37264 ) ;
#16610=PRODUCT_CONTEXT ( 'NONE', #6132, 'mechanical' ) ;
#16656=EDGE_LOOP ( 'NONE', ( #26265, #16945, #37441, #2261 ) ) ;
#16696=PLANE ( 'NONE',  #40974 ) ;
#16747=ORIENTED_EDGE ( 'NONE', *, *, #16315, .T. ) ;
#16762=CARTESIAN_POINT ( 'NONE',  ( -0.4330708661417356775, 0.000000000000000000, 1.186023622047243986 ) ) ;
#16871=DIRECTION ( 'NONE',  ( 0.000000000000000000, -1.000000000000000000, -0.000000000000000000 ) ) ;
#16908=DIRECTION ( 'NONE',  ( 0.000000000000000000, 0.000000000000000000, -1.000000000000000000 ) ) ;
#16945=ORIENTED_EDGE ( 'NONE', *, *, #29891, .F. ) ;
#17036=ORIENTED_EDGE ( 'NONE', *, *, #40135, .T. ) ;
#17044=LINE ( 'NONE', #12994, #21519 ) ;
#17190=CYLINDRICAL_SURFACE ( 'NONE', #22365, 0.1968503937007874405 ) ;
#17242=CIRCLE ( 'NONE', #44009, 0.02900000000000001882 ) ;
#17247=AXIS2_PLACEMENT_3D ( 'NONE', #41305, #8030, #26511 ) ;
#17251=LINE ( 'NONE', #24919, #40787 ) ;
#17273=VERTEX_POINT ( 'NONE', #512 ) ;
#17291=SHAPE_REPRESENTATION ( 'Side Bracket', ( #20860 ), #46110 ) ;
#17444=LINE ( 'NONE', #6414, #32749 ) ;
#17552=DIRECTION ( 'NONE',  ( 0.000000000000000000, 0.000000000000000000, -1.000000000000000000 ) ) ;
#17646=ORIENTED_EDGE ( 'NONE', *, *, #36036, .F. ) ;
#17690=AXIS2_PLACEMENT_3D ( 'NONE', #5659, #5896, #23413 ) ;
#17743=ORIENTED_EDGE ( 'NONE', *, *, #8653, .F. ) ;
#17857=ORIENTED_EDGE ( 'NONE', *, *, #3076, .T. ) ;
#17881=FACE_OUTER_BOUND ( 'NONE', #43686, .T. ) ;
#17889=CARTESIAN_POINT ( 'NONE',  ( 0.2362204724409448231, 0.000000000000000000, 1.186023622047243986 ) ) ;
#17908=EDGE_CURVE ( 'NONE', #35268, #15333, #45208, .T. ) ;
#17921=DIRECTION ( 'NONE',  ( 0.000000000000000000, -1.000000000000000000, 0.000000000000000000 ) ) ;
#18058=VERTEX_POINT ( 'NONE', #14607 ) ;
#18079=AXIS2_PLACEMENT_3D ( 'NONE', #36077, #14752, #9974 ) ;
#18126=ADVANCED_FACE ( 'NONE', ( #40684 ), #12200, .T. ) ;
#18150=ORIENTED_EDGE ( 'NONE', *, *, #14949, .T. ) ;
#18186=EDGE_LOOP ( 'NONE', ( #26826, #10784 ) ) ;
#18244=LINE ( 'NONE', #6982, #46036 ) ;
#18277=ORIENTED_EDGE ( 'NONE', *, *, #10353, .T. ) ;
#18289=PRODUCT_DEFINITION_CONTEXT ( 'detailed design', #37634, 'design' ) ;
#18354=CIRCLE ( 'NONE', #26027, 0.1013779527559055538 ) ;
#18416=ORIENTED_EDGE ( 'NONE', *, *, #21157, .F. ) ;
#18422=CARTESIAN_POINT ( 'NONE',  ( 0.1377952755905511861, 0.1574803149606299191, 0.9074803149606294195 ) ) ;
#18426=DIRECTION ( 'NONE',  ( 0.000000000000000000, 1.000000000000000000, 0.000000000000000000 ) ) ;
#18654=EDGE_CURVE ( 'NONE', #529, #43357, #22915, .T. ) ;
#18799=PLANE ( 'NONE',  #33194 ) ;
#19004=DIRECTION ( 'NONE',  ( -1.000000000000000000, -0.000000000000000000, -0.000000000000000000 ) ) ;
#19016=AXIS2_PLACEMENT_3D ( 'NONE', #40375, #7562, #41073 ) ;
#19033=CYLINDRICAL_SURFACE ( 'NONE', #5202, 0.1624015748031501782 ) ;
#19059=VECTOR ( 'NONE', #21988, 39.37007874015748143 ) ;
#19075=AXIS2_PLACEMENT_3D ( 'NONE', #20850, #2397, #35492 ) ;
#19292=DIRECTION ( 'NONE',  ( -0.000000000000000000, 1.000000000000000000, -0.000000000000000000 ) ) ;
#19298=ORIENTED_EDGE ( 'NONE', *, *, #899, .F. ) ;
#19336=FACE_OUTER_BOUND ( 'NONE', #13795, .T. ) ;
#19359=CONICAL_SURFACE ( 'NONE', #46149, 0.1003937007874010356, 0.7853981633978559529 ) ;
#19362=FACE_OUTER_BOUND ( 'NONE', #20989, .T. ) ;
#19373=DIRECTION ( 'NONE',  ( 1.000000000000000000, 0.000000000000000000, 0.000000000000000000 ) ) ;
#19393=CARTESIAN_POINT ( 'NONE',  ( -0.6195511811023656223, 0.6102362204724408601, 0.5854071585544579071 ) ) ;
#19415=EDGE_LOOP ( 'NONE', ( #11743, #13760, #13306, #30340 ) ) ;
#19504=CARTESIAN_POINT ( 'NONE',  ( -0.6195511811023656223, 0.4133858267716533086, 1.186023622047243986 ) ) ;
#19655=ADVANCED_FACE ( 'NONE', ( #11265, #2693 ), #14214, .T. ) ;
#19689=EDGE_LOOP ( 'NONE', ( #8855, #47161, #6153, #22024 ) ) ;
#19830=LINE ( 'NONE', #34240, #1148 ) ;
#19854=DIRECTION ( 'NONE',  ( 1.000000000000000000, 0.000000000000000000, 0.000000000000000000 ) ) ;
#20073=CARTESIAN_POINT ( 'NONE',  ( -0.4620708661417322616, 0.1864803149606299448, -1.186023622047243986 ) ) ;
#20144=VECTOR ( 'NONE', #6451, 39.37007874015748143 ) ;
#20172=ORIENTED_EDGE ( 'NONE', *, *, #42303, .F. ) ;
#20225=ORIENTED_EDGE ( 'NONE', *, *, #35400, .F. ) ;
#20244=EDGE_CURVE ( 'NONE', #529, #46399, #25336, .T. ) ;
#20280=CARTESIAN_POINT ( 'NONE',  ( -0.6195511811023656223, 1.354170115732555191, -0.4197102375732078561 ) ) ;
#20302=VERTEX_POINT ( 'NONE', #13111 ) ;
#20461=CARTESIAN_POINT ( 'NONE',  ( -0.4620708661417322616, 0.9842519685039375910, -0.8759842519685044904 ) ) ;
#20470=ORIENTED_EDGE ( 'NONE', *, *, #40556, .T. ) ;
#20513=EDGE_CURVE ( 'NONE', #34093, #32371, #42750, .T. ) ;
#20621=EDGE_LOOP ( 'NONE', ( #44647, #39593 ) ) ;
#20722=VECTOR ( 'NONE', #9746, 39.37007874015748143 ) ;
#20734=CARTESIAN_POINT ( 'NONE',  ( -0.6195511811023656223, 1.354170115732555191, -0.4197102375732078561 ) ) ;
#20765=AXIS2_PLACEMENT_3D ( 'NONE', #113, #35624, #2998 ) ;
#20770=EDGE_CURVE ( 'NONE', #13680, #12253, #31569, .T. ) ;
#20772=EDGE_CURVE ( 'NONE', #43655, #44249, #27974, .T. ) ;
#20773=ADVANCED_FACE ( 'NONE', ( #23892 ), #16468, .T. ) ;
#20797=AXIS2_PLACEMENT_3D ( 'NONE', #12815, #23580, #5598 ) ;
#20810=EDGE_LOOP ( 'NONE', ( #40845, #18150 ) ) ;
#20850=CARTESIAN_POINT ( 'NONE',  ( -0.6195511811023656223, 0.000000000000000000, 1.186023622047243986 ) ) ;
#20860=AXIS2_PLACEMENT_3D ( 'NONE', #25692, #32652, #10835 ) ;
#20979=EDGE_CURVE ( 'NONE', #5079, #44357, #26919, .T. ) ;
#20989=EDGE_LOOP ( 'NONE', ( #5941, #11877, #37546, #17743 ) ) ;
#21005=CARTESIAN_POINT ( 'NONE',  ( 0.2362204724409448509, 0.000000000000000000, 0.9891732283464566011 ) ) ;
#21036=ADVANCED_FACE ( 'NONE', ( #6362 ), #35848, .T. ) ;
#21037=ORIENTED_EDGE ( 'NONE', *, *, #21157, .T. ) ;
#21083=PLANE ( 'NONE',  #19075 ) ;
#21157=EDGE_CURVE ( 'NONE', #22637, #42566, #17044, .T. ) ;
#21219=CARTESIAN_POINT ( 'NONE',  ( -0.4330708661417322913, 0.1864803149606299448, -1.186023622047243986 ) ) ;
#21247=FACE_OUTER_BOUND ( 'NONE', #27772, .T. ) ;
#21344=AXIS2_PLACEMENT_3D ( 'NONE', #2106, #34732, #13161 ) ;
#21496=CARTESIAN_POINT ( 'NONE',  ( 0.1377952755905512139, -1.365923996832131609E-16, 0.7066929133858274037 ) ) ;
#21506=CARTESIAN_POINT ( 'NONE',  ( 0.1377952755905511861, 0.1574803149606299191, -0.8070866141732283561 ) ) ;
#21519=VECTOR ( 'NONE', #3124, 39.37007874015748143 ) ;
#21586=EDGE_CURVE ( 'NONE', #15079, #40089, #34604, .T. ) ;
#21597=AXIS2_PLACEMENT_3D ( 'NONE', #23451, #12911, #44978 ) ;
#21709=DIRECTION ( 'NONE',  ( -0.000000000000000000, -0.000000000000000000, 1.000000000000000000 ) ) ;
#21796=CARTESIAN_POINT ( 'NONE',  ( -0.6195511811023656223, 0.9842519685039370358, -0.7135826771653542844 ) ) ;
#21845=DIRECTION ( 'NONE',  ( 0.000000000000000000, 1.000000000000000000, 0.000000000000000000 ) ) ;
#21868=VECTOR ( 'NONE', #16016, 39.37007874015748143 ) ;
#21871=DIRECTION ( 'NONE',  ( 0.000000000000000000, 0.000000000000000000, -1.000000000000000000 ) ) ;
#21914=DIRECTION ( 'NONE',  ( 0.000000000000000000, -1.000000000000000000, 0.000000000000000000 ) ) ;
#21988=DIRECTION ( 'NONE',  ( 1.000000000000000000, -0.000000000000000000, -0.000000000000000000 ) ) ;
#22024=ORIENTED_EDGE ( 'NONE', *, *, #8756, .F. ) ;
#22026=CARTESIAN_POINT ( 'NONE',  ( 0.1377952755905511861, 0.1564960629921262614, -0.8070866141732283561 ) ) ;
#22116=AXIS2_PLACEMENT_3D ( 'NONE', #14748, #37247, #4399 ) ;
#22207=DIRECTION ( 'NONE',  ( 0.000000000000000000, -1.020425574104001164E-16, 1.000000000000000000 ) ) ;
#22221=EDGE_CURVE ( 'NONE', #40227, #42395, #35357, .T. ) ;
#22231=CARTESIAN_POINT ( 'NONE',  ( -0.4620708661417322616, 0.9842519685039375910, -0.5511811023622041894 ) ) ;
#22308=DIRECTION ( 'NONE',  ( 0.000000000000000000, 0.000000000000000000, 1.000000000000000000 ) ) ;
#22365=AXIS2_PLACEMENT_3D ( 'NONE', #21005, #35874, #39453 ) ;
#22427=AXIS2_PLACEMENT_3D ( 'NONE', #3695, #28901, #10911 ) ;
#22437=CARTESIAN_POINT ( 'NONE',  ( 0.4330708661417322913, 0.1574803149606299191, 1.186023622047243986 ) ) ;
#22465=EDGE_CURVE ( 'NONE', #4124, #35796, #30087, .T. ) ;
#22503=ADVANCED_FACE ( 'NONE', ( #24756 ), #44562, .F. ) ;
#22541=VECTOR ( 'NONE', #26765, 39.37007874015748143 ) ;
#22608=AXIS2_PLACEMENT_3D ( 'NONE', #16429, #46103, #2028 ) ;
#22637=VERTEX_POINT ( 'NONE', #7255 ) ;
#22645=CARTESIAN_POINT ( 'NONE',  ( -0.6195511811023656223, 1.354170115732555191, -0.4197102375732078561 ) ) ;
#22652=ORIENTED_EDGE ( 'NONE', *, *, #39484, .F. ) ;
#22697=CYLINDRICAL_SURFACE ( 'NONE', #15258, 0.4724409448818900348 ) ;
#22739=CARTESIAN_POINT ( 'NONE',  ( -0.4620708661417322616, 0.000000000000000000, -1.186023622047243986 ) ) ;
#22755=ORIENTED_EDGE ( 'NONE', *, *, #37677, .T. ) ;
#22833=CARTESIAN_POINT ( 'NONE',  ( -0.4330708661417356775, 0.000000000000000000, -1.186023622047243986 ) ) ;
#22915=LINE ( 'NONE', #22437, #33050 ) ;
#22924=CARTESIAN_POINT ( 'NONE',  ( -0.6195511811023656223, 0.6102362204724408601, 0.5167322834645649010 ) ) ;
#22934=VECTOR ( 'NONE', #16871, 39.37007874015748143 ) ;
#22995=AXIS2_PLACEMENT_3D ( 'NONE', #11733, #26352, #23217 ) ;
#23078=CARTESIAN_POINT ( 'NONE',  ( -0.4330708661417356775, 0.1864803149606299171, -1.186023622047243986 ) ) ;
#23079=ORIENTED_EDGE ( 'NONE', *, *, #1300, .F. ) ;
#23121=ORIENTED_EDGE ( 'NONE', *, *, #27183, .T. ) ;
#23217=DIRECTION ( 'NONE',  ( 0.000000000000000000, 0.000000000000000000, -1.000000000000000000 ) ) ;
#23264=EDGE_CURVE ( 'NONE', #2549, #43655, #8581, .T. ) ;
#23413=DIRECTION ( 'NONE',  ( -8.673617379884034486E-16, 0.000000000000000000, -1.000000000000000000 ) ) ;
#23437=AXIS2_PLACEMENT_3D ( 'NONE', #7700, #44343, #8167 ) ;
#23451=CARTESIAN_POINT ( 'NONE',  ( 0.1377952755905511861, 0.1564960629921262614, -0.8070866141732283561 ) ) ;
#23466=CARTESIAN_POINT ( 'NONE',  ( -0.6195511811023656223, 0.6102362204724407491, 0.9891732283464566011 ) ) ;
#23468=CYLINDRICAL_SURFACE ( 'NONE', #10032, 0.1968503937007874405 ) ;
#23580=DIRECTION ( 'NONE',  ( 0.000000000000000000, 1.000000000000000000, 0.000000000000000000 ) ) ;
#23638=ORIENTED_EDGE ( 'NONE', *, *, #3076, .F. ) ;
#23755=ORIENTED_EDGE ( 'NONE', *, *, #26876, .T. ) ;
#23892=FACE_OUTER_BOUND ( 'NONE', #36930, .T. ) ;
#23894=CARTESIAN_POINT ( 'NONE',  ( 0.1377952755905511861, 0.1564960629921262614, 0.8070866141732283561 ) ) ;
#24082=EDGE_LOOP ( 'NONE', ( #30690, #26509, #13748, #47356, #34429, #25572, #24393, #35162 ) ) ;
#24088=PLANE ( 'NONE',  #22608 ) ;
#24316=VECTOR ( 'NONE', #31788, 39.37007874015748143 ) ;
#24332=AXIS2_PLACEMENT_3D ( 'NONE', #8001, #30332, #41270 ) ;
#24349=EDGE_LOOP ( 'NONE', ( #42929, #127, #31924, #24644 ) ) ;
#24362=FACE_OUTER_BOUND ( 'NONE', #11827, .T. ) ;
#24375=ORIENTED_EDGE ( 'NONE', *, *, #26702, .T. ) ;
#24393=ORIENTED_EDGE ( 'NONE', *, *, #40983, .F. ) ;
#24432=LINE ( 'NONE', #28053, #39425 ) ;
#24436=VERTEX_POINT ( 'NONE', #37806 ) ;
#24538=CARTESIAN_POINT ( 'NONE',  ( 0.2362204724409448509, 0.000000000000000000, -1.186023622047243986 ) ) ;
#24541=ORIENTED_EDGE ( 'NONE', *, *, #2905, .T. ) ;
#24619=ORIENTED_EDGE ( 'NONE', *, *, #37677, .F. ) ;
#24644=ORIENTED_EDGE ( 'NONE', *, *, #46577, .F. ) ;
#24668=DIMENSIONAL_EXPONENTS ( 1.000000000000000000, 0.000000000000000000, 0.000000000000000000, 0.000000000000000000, 0.000000000000000000, 0.000000000000000000, 0.000000000000000000 ) ;
#24674=AXIS2_PLACEMENT_3D ( 'NONE', #4101, #3645, #26 ) ;
#24705=EDGE_CURVE ( 'NONE', #37245, #35268, #17251, .T. ) ;
#24727=EDGE_CURVE ( 'NONE', #18058, #5079, #39043, .T. ) ;
#24756=FACE_OUTER_BOUND ( 'NONE', #19689, .T. ) ;
#24826=ORIENTED_EDGE ( 'NONE', *, *, #47238, .T. ) ;
#24919=CARTESIAN_POINT ( 'NONE',  ( 0.1377952755905511861, 0.1574803149606299191, -0.7066929133858274037 ) ) ;
#24928=CARTESIAN_POINT ( 'NONE',  ( 0.1377952755905511861, -1.365923996832131609E-16, -0.7066929133858274037 ) ) ;
#24965=CIRCLE ( 'NONE', #23437, 0.1003937007874010356 ) ;
#25011=ADVANCED_FACE ( 'NONE', ( #4484, #44054 ), #14602, .F. ) ;
#25085=VERTEX_POINT ( 'NONE', #29734 ) ;
#25116=VECTOR ( 'NONE', #1632, 39.37007874015748143 ) ;
#25136=EDGE_LOOP ( 'NONE', ( #27573, #28332, #9633, #45277 ) ) ;
#25149=CIRCLE ( 'NONE', #4455, 0.4724409448818900348 ) ;
#25210=EDGE_CURVE ( 'NONE', #17273, #42395, #33787, .T. ) ;
#25244=CARTESIAN_POINT ( 'NONE',  ( 0.1377952755905511861, 0.1564960629921262614, -0.7066929133858274037 ) ) ;
#25258=VECTOR ( 'NONE', #17921, 39.37007874015748143 ) ;
#25336=CIRCLE ( 'NONE', #17690, 0.1968503937007874405 ) ;
#25355=DIRECTION ( 'NONE',  ( 1.000000000000000000, -0.000000000000000000, -0.000000000000000000 ) ) ;
#25483=DIRECTION ( 'NONE',  ( 0.000000000000000000, -1.000000000000000000, 0.000000000000000000 ) ) ;
#25560=CARTESIAN_POINT ( 'NONE',  ( 0.4330708661417322913, 0.1574803149606299191, -0.9891732283464564901 ) ) ;
#25572=ORIENTED_EDGE ( 'NONE', *, *, #40135, .F. ) ;
#25628=ORIENTED_EDGE ( 'NONE', *, *, #33855, .T. ) ;
#25648=CARTESIAN_POINT ( 'NONE',  ( -0.6195511811023656223, 0.9842519685039370358, -1.186023622047243986 ) ) ;
#25692=CARTESIAN_POINT ( 'NONE',  ( 0.000000000000000000, 0.000000000000000000, 0.000000000000000000 ) ) ;
#25793=ORIENTED_EDGE ( 'NONE', *, *, #30410, .T. ) ;
#25825=EDGE_CURVE ( 'NONE', #27278, #40074, #26297, .T. ) ;
#25972=CIRCLE ( 'NONE', #5294, 0.1013779527559055538 ) ;
#26027=AXIS2_PLACEMENT_3D ( 'NONE', #2716, #4711, #42011 ) ;
#26067=DIRECTION ( 'NONE',  ( 0.000000000000000000, 1.000000000000000000, 0.000000000000000000 ) ) ;
#26171=FILL_AREA_STYLE_COLOUR ( '', #13215 ) ;
#26265=ORIENTED_EDGE ( 'NONE', *, *, #6011, .F. ) ;
#26297=LINE ( 'NONE', #40854, #22541 ) ;
#26300=PRODUCT_DEFINITION_FORMATION_WITH_SPECIFIED_SOURCE ( 'ANY', '', #14590, .NOT_KNOWN. ) ;
#26352=DIRECTION ( 'NONE',  ( 1.000000000000000000, -0.000000000000000000, -0.000000000000000000 ) ) ;
#26412=FILL_AREA_STYLE ('',( #26171 ) ) ;
#26461=CARTESIAN_POINT ( 'NONE',  ( 0.4330708661417322913, 0.000000000000000000, -1.186023622047243986 ) ) ;
#26509=ORIENTED_EDGE ( 'NONE', *, *, #21586, .T. ) ;
#26511=DIRECTION ( 'NONE',  ( 0.000000000000000000, 0.000000000000000000, -1.000000000000000000 ) ) ;
#26672=DIRECTION ( 'NONE',  ( 0.000000000000000000, 0.000000000000000000, -1.000000000000000000 ) ) ;
#26702=EDGE_CURVE ( 'NONE', #5079, #32371, #4496, .T. ) ;
#26765=DIRECTION ( 'NONE',  ( -0.000000000000000000, 0.000000000000000000, 1.000000000000000000 ) ) ;
#26814=VECTOR ( 'NONE', #39717, 39.37007874015748143 ) ;
#26826=ORIENTED_EDGE ( 'NONE', *, *, #39484, .T. ) ;
#26832=DIRECTION ( 'NONE',  ( 1.000000000000000000, 0.000000000000000000, 0.000000000000000000 ) ) ;
#26876=EDGE_CURVE ( 'NONE', #43147, #37245, #41910, .T. ) ;
#26881=AXIS2_PLACEMENT_3D ( 'NONE', #27277, #34926, #41827 ) ;
#26911=ORIENTED_EDGE ( 'NONE', *, *, #42538, .F. ) ;
#26919=CIRCLE ( 'NONE', #13892, 0.02900000000000001882 ) ;
#26997=ORIENTED_EDGE ( 'NONE', *, *, #30136, .T. ) ;
#27097=ORIENTED_EDGE ( 'NONE', *, *, #39010, .F. ) ;
#27138=EDGE_CURVE ( 'NONE', #40089, #4124, #42359, .T. ) ;
#27177=CARTESIAN_POINT ( 'NONE',  ( 0.1377952755905512139, 0.1574803149606299191, 0.7057086614173228023 ) ) ;
#27183=EDGE_CURVE ( 'NONE', #29873, #37690, #8833, .T. ) ;
#27277=CARTESIAN_POINT ( 'NONE',  ( -0.6195511811023656223, 0.6102362204724408601, 0.5167322834645649010 ) ) ;
#27278=VERTEX_POINT ( 'NONE', #10502 ) ;
#27573=ORIENTED_EDGE ( 'NONE', *, *, #31586, .F. ) ;
#27710=DIRECTION ( 'NONE',  ( -0.000000000000000000, 1.000000000000000000, -0.000000000000000000 ) ) ;
#27766=ORIENTED_EDGE ( 'NONE', *, *, #27183, .F. ) ;
#27772=EDGE_LOOP ( 'NONE', ( #3624, #13933, #892, #14164 ) ) ;
#27798=DIRECTION ( 'NONE',  ( 0.000000000000000000, 0.000000000000000000, -1.000000000000000000 ) ) ;
#27974=LINE ( 'NONE', #34686, #60 ) ;
#27988=ORIENTED_EDGE ( 'NONE', *, *, #9307, .T. ) ;
#27996=ORIENTED_EDGE ( 'NONE', *, *, #7622, .T. ) ;
#28053=CARTESIAN_POINT ( 'NONE',  ( 0.1377952755905511861, 0.1564960629921262614, -0.7066929133858274037 ) ) ;
#28137=CARTESIAN_POINT ( 'NONE',  ( 0.1377952755905511861, 0.1564960629921262614, -0.8070866141732283561 ) ) ;
#28196=FACE_BOUND ( 'NONE', #20810, .T. ) ;
#28199=DIRECTION ( 'NONE',  ( 1.000000000000000000, 0.000000000000000000, 0.000000000000000000 ) ) ;
#28332=ORIENTED_EDGE ( 'NONE', *, *, #25825, .F. ) ;
#28438=EDGE_CURVE ( 'NONE', #20302, #6854, #12190, .T. ) ;
#28585=( GEOMETRIC_REPRESENTATION_CONTEXT ( 3 ) GLOBAL_UNCERTAINTY_ASSIGNED_CONTEXT ( ( #4897 ) ) GLOBAL_UNIT_ASSIGNED_CONTEXT ( ( #37648, #11794, #34311 ) ) REPRESENTATION_CONTEXT ( 'NONE', 'WORKASPACE' ) ) ;
#28589=VECTOR ( 'NONE', #19004, 39.37007874015748143 ) ;
#28650=CYLINDRICAL_SURFACE ( 'NONE', #33123, 0.02900000000000001882 ) ;
#28737=VECTOR ( 'NONE', #11597, 39.37007874015748143 ) ;
#28744=FACE_OUTER_BOUND ( 'NONE', #16656, .T. ) ;
#28893=EDGE_CURVE ( 'NONE', #24436, #46224, #25972, .T. ) ;
#28901=DIRECTION ( 'NONE',  ( 0.000000000000000000, -1.000000000000000000, 0.000000000000000000 ) ) ;
#28983=DIRECTION ( 'NONE',  ( 0.000000000000000000, 0.000000000000000000, 1.000000000000000000 ) ) ;
#28989=DIRECTION ( 'NONE',  ( 0.000000000000000000, 0.000000000000000000, 1.000000000000000000 ) ) ;
#28991=ORIENTED_EDGE ( 'NONE', *, *, #40983, .T. ) ;
#29020=DIRECTION ( 'NONE',  ( -0.000000000000000000, 1.000000000000000000, -0.000000000000000000 ) ) ;
#29063=ORIENTED_EDGE ( 'NONE', *, *, #23264, .T. ) ;
#29092=LINE ( 'NONE', #43170, #32319 ) ;
#29108=CARTESIAN_POINT ( 'NONE',  ( -0.4620708661417322616, 0.4133858267716533086, 0.9891732283464566011 ) ) ;
#29131=CIRCLE ( 'NONE', #32166, 0.1003937007874010356 ) ;
#29134=EDGE_LOOP ( 'NONE', ( #17646, #9992, #27766, #24826, #28991, #32217, #9643, #33538 ) ) ;
#29200=CYLINDRICAL_SURFACE ( 'NONE', #19016, 0.1968503937007874405 ) ;
#29243=UNCERTAINTY_MEASURE_WITH_UNIT (LENGTH_MEASURE( 1.000000000000000082E-05 ), #30026, 'distance_accuracy_value', 'NONE') ;
#29249=VECTOR ( 'NONE', #30838, 39.37007874015748143 ) ;
#29395=ADVANCED_FACE ( 'NONE', ( #9377, #42169, #35263 ), #21083, .T. ) ;
#29414=LINE ( 'NONE', #11859, #16189 ) ;
#29482=VECTOR ( 'NONE', #40921, 39.37007874015748143 ) ;
#29565=( NAMED_UNIT ( * ) PLANE_ANGLE_UNIT ( ) SI_UNIT ( $, .RADIAN. ) ) ;
#29734=CARTESIAN_POINT ( 'NONE',  ( -0.6195511811023656223, 0.6529540528279709211, 0.4629603087243971959 ) ) ;
#29743=CARTESIAN_POINT ( 'NONE',  ( 0.1377952755905511861, -1.365923996832131609E-16, -0.8070866141732283561 ) ) ;
#29845=LINE ( 'NONE', #26461, #37110 ) ;
#29851=CARTESIAN_POINT ( 'NONE',  ( 0.4330708661417322913, 0.1574803149606299191, 0.9891732283464566011 ) ) ;
#29868=CARTESIAN_POINT ( 'NONE',  ( -0.4620708661417322616, 0.6102362204724407491, 1.186023622047243986 ) ) ;
#29873=VERTEX_POINT ( 'NONE', #37606 ) ;
#29883=VERTEX_POINT ( 'NONE', #19393 ) ;
#29891=EDGE_CURVE ( 'NONE', #37245, #43147, #35956, .T. ) ;
#29969=FACE_OUTER_BOUND ( 'NONE', #1835, .T. ) ;
#29994=VERTEX_POINT ( 'NONE', #9573 ) ;
#30026=( CONVERSION_BASED_UNIT ( 'INCH', #7228 ) LENGTH_UNIT ( ) NAMED_UNIT ( #39334 ) ) ;
#30055=CARTESIAN_POINT ( 'NONE',  ( -0.6195511811023656223, 0.9842519685039375910, -0.7135826771653542844 ) ) ;
#30062=CARTESIAN_POINT ( 'NONE',  ( -0.6195511811023656223, 0.4133858267716533086, 1.186023622047243986 ) ) ;
#30087=CIRCLE ( 'NONE', #32361, 0.1968503937007874405 ) ;
#30136=EDGE_CURVE ( 'NONE', #43357, #20302, #10274, .T. ) ;
#30204=DIRECTION ( 'NONE',  ( 0.000000000000000000, 0.000000000000000000, -1.000000000000000000 ) ) ;
#30238=ADVANCED_FACE ( 'NONE', ( #6658 ), #14343, .F. ) ;
#30262=CYLINDRICAL_SURFACE ( 'NONE', #2735, 0.1003937007874010356 ) ;
#30308=LINE ( 'NONE', #44859, #28737 ) ;
#30332=DIRECTION ( 'NONE',  ( 0.000000000000000000, 1.000000000000000000, 0.000000000000000000 ) ) ;
#30340=ORIENTED_EDGE ( 'NONE', *, *, #16315, .F. ) ;
#30374=LINE ( 'NONE', #44921, #29249 ) ;
#30410=EDGE_CURVE ( 'NONE', #42395, #40227, #29131, .T. ) ;
#30489=SURFACE_STYLE_USAGE ( .BOTH. , #12510 ) ;
#30515=ORIENTED_EDGE ( 'NONE', *, *, #42303, .T. ) ;
#30634=ORIENTED_EDGE ( 'NONE', *, *, #44495, .T. ) ;
#30651=EDGE_CURVE ( 'NONE', #15079, #40074, #34923, .T. ) ;
#30690=ORIENTED_EDGE ( 'NONE', *, *, #30651, .F. ) ;
#30693=EDGE_LOOP ( 'NONE', ( #26911, #35743, #34046, #27988, #23121, #41368 ) ) ;
#30834=ORIENTED_EDGE ( 'NONE', *, *, #42538, .T. ) ;
#30838=DIRECTION ( 'NONE',  ( 0.000000000000000000, -0.6220299971367094782, 0.7829934116339072325 ) ) ;
#30879=ORIENTED_EDGE ( 'NONE', *, *, #20770, .F. ) ;
#30887=MECHANICAL_DESIGN_GEOMETRIC_PRESENTATION_REPRESENTATION('',(#43806),#28585);
#31273=FACE_OUTER_BOUND ( 'NONE', #42823, .T. ) ;
#31292=ADVANCED_FACE ( 'NONE', ( #29969 ), #44516, .F. ) ;
#31325=DIRECTION ( 'NONE',  ( 0.000000000000000000, -0.000000000000000000, -1.000000000000000000 ) ) ;
#31468=CARTESIAN_POINT ( 'NONE',  ( -0.4620708661417322616, 0.6102362204724407491, 0.9891732283464566011 ) ) ;
#31569=LINE ( 'NONE', #20280, #20722 ) ;
#31586=EDGE_CURVE ( 'NONE', #40074, #12155, #8475, .T. ) ;
#31721=CARTESIAN_POINT ( 'NONE',  ( -0.4620708661417322616, 0.9842519685039370358, -0.7135826771653542844 ) ) ;
#31762=ADVANCED_FACE ( 'NONE', ( #8834 ), #23468, .T. ) ;
#31788=DIRECTION ( 'NONE',  ( 0.000000000000000000, -0.6220299971367094782, 0.7829934116339072325 ) ) ;
#31803=LINE ( 'NONE', #13564, #33672 ) ;
#31857=CARTESIAN_POINT ( 'NONE',  ( 0.1377952755905511861, -1.365923996832131609E-16, -0.8070866141732283561 ) ) ;
#31880=ADVANCED_BREP_SHAPE_REPRESENTATION ( 'Side Bracket', ( #37046, #20860 ), #46110 ) ;
#31924=ORIENTED_EDGE ( 'NONE', *, *, #20244, .F. ) ;
#31926=ORIENTED_EDGE ( 'NONE', *, *, #6259, .F. ) ;
#32030=ORIENTED_EDGE ( 'NONE', *, *, #1873, .T. ) ;
#32075=DIRECTION ( 'NONE',  ( 0.000000000000000000, 1.000000000000000000, 0.000000000000000000 ) ) ;
#32085=EDGE_LOOP ( 'NONE', ( #32030, #3854, #21037, #30634, #23638, #22755, #44775, #8193 ) ) ;
#32166=AXIS2_PLACEMENT_3D ( 'NONE', #4705, #26067, #40636 ) ;
#32217=ORIENTED_EDGE ( 'NONE', *, *, #20513, .T. ) ;
#32231=ORIENTED_EDGE ( 'NONE', *, *, #33256, .F. ) ;
#32319=VECTOR ( 'NONE', #13957, 39.37007874015748143 ) ;
#32360=AXIS2_PLACEMENT_3D ( 'NONE', #23078, #1969, #12551 ) ;
#32361=AXIS2_PLACEMENT_3D ( 'NONE', #29108, #9681, #42937 ) ;
#32371=VERTEX_POINT ( 'NONE', #13729 ) ;
#32627=ORIENTED_EDGE ( 'NONE', *, *, #20772, .F. ) ;
#32652=DIRECTION ( 'NONE',  ( 0.000000000000000000, 0.000000000000000000, 1.000000000000000000 ) ) ;
#32749=VECTOR ( 'NONE', #10270, 39.37007874015748143 ) ;
#32827=ORIENTED_EDGE ( 'NONE', *, *, #6381, .F. ) ;
#32829=ORIENTED_EDGE ( 'NONE', *, *, #3183, .F. ) ;
#32837=DIRECTION ( 'NONE',  ( -0.000000000000000000, 1.000000000000000000, -0.000000000000000000 ) ) ;
#33010=AXIS2_PLACEMENT_3D ( 'NONE', #44993, #37840, #26832 ) ;
#33041=ORIENTED_EDGE ( 'NONE', *, *, #23264, .F. ) ;
#33050=VECTOR ( 'NONE', #143, 39.37007874015748143 ) ;
#33123=AXIS2_PLACEMENT_3D ( 'NONE', #43209, #39619, #36045 ) ;
#33194=AXIS2_PLACEMENT_3D ( 'NONE', #22645, #8253, #351 ) ;
#33256=EDGE_CURVE ( 'NONE', #40227, #46224, #29092, .T. ) ;
#33360=CIRCLE ( 'NONE', #5034, 0.1003937007874010356 ) ;
#33503=LINE ( 'NONE', #22924, #6242 ) ;
#33538=ORIENTED_EDGE ( 'NONE', *, *, #20979, .T. ) ;
#33560=ORIENTED_EDGE ( 'NONE', *, *, #21586, .F. ) ;
#33672=VECTOR ( 'NONE', #28199, 39.37007874015748143 ) ;
#33787=LINE ( 'NONE', #18422, #260 ) ;
#33811=AXIS2_PLACEMENT_3D ( 'NONE', #8585, #34026, #19373 ) ;
#33855=EDGE_CURVE ( 'NONE', #29883, #40089, #33503, .T. ) ;
#34026=DIRECTION ( 'NONE',  ( -0.000000000000000000, 0.000000000000000000, 1.000000000000000000 ) ) ;
#34046=ORIENTED_EDGE ( 'NONE', *, *, #1873, .F. ) ;
#34082=SURFACE_STYLE_FILL_AREA ( #26412 ) ;
#34093=VERTEX_POINT ( 'NONE', #25648 ) ;
#34151=DIRECTION ( 'NONE',  ( -1.000000000000000000, -0.000000000000000000, -0.000000000000000000 ) ) ;
#34240=CARTESIAN_POINT ( 'NONE',  ( -0.4620708661417322616, 0.6102362204724408601, 0.5167322834645649010 ) ) ;
#34310=VECTOR ( 'NONE', #43669, 39.37007874015748143 ) ;
#34311=( NAMED_UNIT ( * ) SI_UNIT ( $, .STERADIAN. ) SOLID_ANGLE_UNIT ( ) ) ;
#34429=ORIENTED_EDGE ( 'NONE', *, *, #10628, .F. ) ;
#34604=CIRCLE ( 'NONE', #13934, 0.1968503937007874405 ) ;
#34625=PLANE ( 'NONE',  #1243 ) ;
#34645=CONICAL_SURFACE ( 'NONE', #21597, 0.1003937007874010356, 0.7853981633978559529 ) ;
#34686=CARTESIAN_POINT ( 'NONE',  ( -0.4620708661417322616, 0.9842519685039375910, -0.5511811023622041894 ) ) ;
#34732=DIRECTION ( 'NONE',  ( 0.000000000000000000, -1.000000000000000000, 0.000000000000000000 ) ) ;
#34835=SHAPE_DEFINITION_REPRESENTATION ( #43248, #17291 ) ;
#34857=CARTESIAN_POINT ( 'NONE',  ( 0.2362204724409448231, 0.000000000000000000, -1.186023622047243986 ) ) ;
#34923=LINE ( 'NONE', #42318, #43603 ) ;
#34926=DIRECTION ( 'NONE',  ( -0.000000000000000000, 1.000000000000000000, 1.020425574104001164E-16 ) ) ;
#34957=ORIENTED_EDGE ( 'NONE', *, *, #11424, .T. ) ;
#35149=DIRECTION ( 'NONE',  ( 0.000000000000000000, -1.000000000000000000, 0.000000000000000000 ) ) ;
#35162=ORIENTED_EDGE ( 'NONE', *, *, #25825, .T. ) ;
#35169=CIRCLE ( 'NONE', #22116, 0.1968503937007874405 ) ;
#35263=FACE_OUTER_BOUND ( 'NONE', #30693, .T. ) ;
#35268=VERTEX_POINT ( 'NONE', #25244 ) ;
#35339=ORIENTED_EDGE ( 'NONE', *, *, #22221, .F. ) ;
#35357=CIRCLE ( 'NONE', #20797, 0.1003937007874010356 ) ;
#35400=EDGE_CURVE ( 'NONE', #43655, #2549, #5572, .T. ) ;
#35492=DIRECTION ( 'NONE',  ( 0.000000000000000000, -0.000000000000000000, -1.000000000000000000 ) ) ;
#35583=VECTOR ( 'NONE', #34151, 39.37007874015748143 ) ;
#35624=DIRECTION ( 'NONE',  ( -0.000000000000000000, 0.000000000000000000, 1.000000000000000000 ) ) ;
#35743=ORIENTED_EDGE ( 'NONE', *, *, #28438, .T. ) ;
#35750=ORIENTED_EDGE ( 'NONE', *, *, #26876, .F. ) ;
#35796=VERTEX_POINT ( 'NONE', #38990 ) ;
#35823=ADVANCED_FACE ( 'NONE', ( #7294 ), #36536, .T. ) ;
#35848=PLANE ( 'NONE',  #20765 ) ;
#35874=DIRECTION ( 'NONE',  ( 0.000000000000000000, 1.000000000000000000, 0.000000000000000000 ) ) ;
#35882=EDGE_CURVE ( 'NONE', #37690, #44293, #43084, .T. ) ;
#35956=CIRCLE ( 'NONE', #44377, 0.1003937007874010356 ) ;
#36036=EDGE_CURVE ( 'NONE', #46399, #44357, #4374, .T. ) ;
#36045=DIRECTION ( 'NONE',  ( 1.000000000000000000, 0.000000000000000000, 0.000000000000000000 ) ) ;
#36077=CARTESIAN_POINT ( 'NONE',  ( -0.4620708661417322616, 0.9842519685039370358, -0.7135826771653542844 ) ) ;
#36103=ORIENTED_EDGE ( 'NONE', *, *, #7622, .F. ) ;
#36140=AXIS2_PLACEMENT_3D ( 'NONE', #28137, #6533, #43420 ) ;
#36141=FACE_OUTER_BOUND ( 'NONE', #12600, .T. ) ;
#36154=ORIENTED_EDGE ( 'NONE', *, *, #39010, .T. ) ;
#36435=AXIS2_PLACEMENT_3D ( 'NONE', #21506, #43065, #47156 ) ;
#36536=CYLINDRICAL_SURFACE ( 'NONE', #22427, 0.1968503937007874405 ) ;
#36930=EDGE_LOOP ( 'NONE', ( #25628, #43011, #20172, #24541 ) ) ;
#37046=MANIFOLD_SOLID_BREP ( 'Side Bracket', #41538 ) ;
#37079=VECTOR ( 'NONE', #6289, 39.37007874015748143 ) ;
#37110=VECTOR ( 'NONE', #44163, 39.37007874015748143 ) ;
#37154=CIRCLE ( 'NONE', #17247, 0.1624015748031501782 ) ;
#37245=VERTEX_POINT ( 'NONE', #24928 ) ;
#37247=DIRECTION ( 'NONE',  ( -1.000000000000000000, -0.000000000000000000, -0.000000000000000000 ) ) ;
#37264=DIRECTION ( 'NONE',  ( 0.000000000000000000, 0.000000000000000000, -1.000000000000000000 ) ) ;
#37295=CARTESIAN_POINT ( 'NONE',  ( -0.4620708661417322616, 0.9842519685039375910, -0.8759842519685044904 ) ) ;
#37441=ORIENTED_EDGE ( 'NONE', *, *, #24705, .T. ) ;
#37462=CARTESIAN_POINT ( 'NONE',  ( -0.6195511811023656223, 0.9842519685039375910, -0.5511811023622041894 ) ) ;
#37512=ORIENTED_EDGE ( 'NONE', *, *, #10628, .T. ) ;
#37546=ORIENTED_EDGE ( 'NONE', *, *, #8756, .T. ) ;
#37606=CARTESIAN_POINT ( 'NONE',  ( -0.4330708661417356775, 0.000000000000000000, -1.186023622047243986 ) ) ;
#37634=APPLICATION_CONTEXT ( 'automotive_design' ) ;
#37648=( CONVERSION_BASED_UNIT ( 'INCH', #41442 ) LENGTH_UNIT ( ) NAMED_UNIT ( #24668 ) ) ;
#37677=EDGE_CURVE ( 'NONE', #35796, #15079, #4878, .T. ) ;
#37690=VERTEX_POINT ( 'NONE', #34857 ) ;
#37806=CARTESIAN_POINT ( 'NONE',  ( 0.1377952755905511861, 0.1574803149606299191, 0.9084645669291339098 ) ) ;
#37840=DIRECTION ( 'NONE',  ( -0.000000000000000000, 0.000000000000000000, 1.000000000000000000 ) ) ;
#37974=DIRECTION ( 'NONE',  ( 0.000000000000000000, 0.000000000000000000, -1.000000000000000000 ) ) ;
#38047=ORIENTED_EDGE ( 'NONE', *, *, #6011, .T. ) ;
#38153=VECTOR ( 'NONE', #5743, 39.37007874015748143 ) ;
#38184=DIRECTION ( 'NONE',  ( 0.000000000000000000, 0.000000000000000000, -1.000000000000000000 ) ) ;
#38204=DIRECTION ( 'NONE',  ( 0.000000000000000000, 0.000000000000000000, 1.000000000000000000 ) ) ;
#38327=CARTESIAN_POINT ( 'NONE',  ( -0.4620708661417322616, 1.354170115732555191, -0.4197102375732078561 ) ) ;
#38425=ADVANCED_FACE ( 'NONE', ( #28744 ), #10513, .F. ) ;
#38575=CARTESIAN_POINT ( 'NONE',  ( 0.1377952755905512139, 0.1564960629921262614, -0.9074803149606294195 ) ) ;
#38802=ADVANCED_FACE ( 'NONE', ( #28196, #42535, #1826 ), #16696, .F. ) ;
#38990=CARTESIAN_POINT ( 'NONE',  ( -0.4620708661417322616, 0.4133858267716533086, 1.186023622047243986 ) ) ;
#39010=EDGE_CURVE ( 'NONE', #32371, #12253, #47167, .T. ) ;
#39043=LINE ( 'NONE', #13889, #20144 ) ;
#39113=CARTESIAN_POINT ( 'NONE',  ( -0.6195511811023656223, 0.000000000000000000, -1.186023622047243986 ) ) ;
#39150=ORIENTED_EDGE ( 'NONE', *, *, #22221, .T. ) ;
#39205=ADVANCED_FACE ( 'NONE', ( #31273 ), #34625, .F. ) ;
#39256=AXIS2_PLACEMENT_3D ( 'NONE', #5702, #21914, #46181 ) ;
#39334=DIMENSIONAL_EXPONENTS ( 1.000000000000000000, 0.000000000000000000, 0.000000000000000000, 0.000000000000000000, 0.000000000000000000, 0.000000000000000000, 0.000000000000000000 ) ;
#39425=VECTOR ( 'NONE', #2607, 39.37007874015748143 ) ;
#39453=DIRECTION ( 'NONE',  ( 0.000000000000000000, 0.000000000000000000, 1.000000000000000000 ) ) ;
#39474=ADVANCED_FACE ( 'NONE', ( #1436 ), #30262, .F. ) ;
#39482=CARTESIAN_POINT ( 'NONE',  ( 0.1377952755905511861, 0.1574803149606299191, -0.8070866141732283561 ) ) ;
#39484=EDGE_CURVE ( 'NONE', #17273, #3953, #24965, .T. ) ;
#39593=ORIENTED_EDGE ( 'NONE', *, *, #8653, .T. ) ;
#39619=DIRECTION ( 'NONE',  ( -0.000000000000000000, 0.000000000000000000, 1.000000000000000000 ) ) ;
#39696=AXIS2_PLACEMENT_3D ( 'NONE', #1038, #15696, #38184 ) ;
#39717=DIRECTION ( 'NONE',  ( -0.000000000000000000, 1.000000000000000000, -0.000000000000000000 ) ) ;
#39860=EDGE_CURVE ( 'NONE', #16170, #43692, #45033, .T. ) ;
#40074=VERTEX_POINT ( 'NONE', #45887 ) ;
#40089=VERTEX_POINT ( 'NONE', #1811 ) ;
#40135=EDGE_CURVE ( 'NONE', #34093, #13680, #25149, .T. ) ;
#40227=VERTEX_POINT ( 'NONE', #43468 ) ;
#40375=CARTESIAN_POINT ( 'NONE',  ( -0.6195511811023656223, 0.8070866141732282451, 0.5854071585544579071 ) ) ;
#40457=DIRECTION ( 'NONE',  ( -0.000000000000000000, 1.000000000000000000, -0.000000000000000000 ) ) ;
#40503=SHAPE_REPRESENTATION_RELATIONSHIP ( 'NONE' , 'NONE' ,  #17291, #31880 ) ;
#40544=AXIS2_PLACEMENT_3D ( 'NONE', #39482, #3054, #28989 ) ;
#40556=EDGE_CURVE ( 'NONE', #15333, #35268, #12098, .T. ) ;
#40636=DIRECTION ( 'NONE',  ( 0.000000000000000000, 0.000000000000000000, -1.000000000000000000 ) ) ;
#40684=FACE_OUTER_BOUND ( 'NONE', #25136, .T. ) ;
#40787=VECTOR ( 'NONE', #29020, 39.37007874015748143 ) ;
#40845=ORIENTED_EDGE ( 'NONE', *, *, #28893, .T. ) ;
#40854=CARTESIAN_POINT ( 'NONE',  ( -0.6195511811023656223, 0.1864803149606299171, 1.186023622047243986 ) ) ;
#40921=DIRECTION ( 'NONE',  ( 0.000000000000000000, 1.000000000000000000, 0.000000000000000000 ) ) ;
#40974=AXIS2_PLACEMENT_3D ( 'NONE', #41821, #35149, #31325 ) ;
#40983=EDGE_CURVE ( 'NONE', #27278, #34093, #9905, .T. ) ;
#41016=LINE ( 'NONE', #22833, #1938 ) ;
#41058=FACE_OUTER_BOUND ( 'NONE', #2834, .T. ) ;
#41073=DIRECTION ( 'NONE',  ( 0.000000000000000000, 0.000000000000000000, 1.000000000000000000 ) ) ;
#41270=DIRECTION ( 'NONE',  ( 0.000000000000000000, 0.000000000000000000, -1.000000000000000000 ) ) ;
#41305=CARTESIAN_POINT ( 'NONE',  ( -0.4620708661417322616, 0.9842519685039375910, -0.7135826771653542844 ) ) ;
#41368=ORIENTED_EDGE ( 'NONE', *, *, #35882, .T. ) ;
#41442=LENGTH_MEASURE_WITH_UNIT ( LENGTH_MEASURE( 0.02539999999999999897 ), #5051 ) ;
#41538=CLOSED_SHELL ( 'NONE', ( #22503, #2639, #11221, #39474, #30238, #1356, #6442, #29395, #21036, #20773, #130, #25011, #19655, #38802, #39205, #38425, #4526, #31292, #523, #46828, #47062, #18126, #46999, #35823, #31762, #13645 ) ) ;
#41604=CARTESIAN_POINT ( 'NONE',  ( 0.1377952755905511861, 0.1564960629921262614, 0.9074803149606294195 ) ) ;
#41675=DIRECTION ( 'NONE',  ( 0.000000000000000000, 0.000000000000000000, 1.000000000000000000 ) ) ;
#41786=CARTESIAN_POINT ( 'NONE',  ( 0.1377952755905511861, -1.365923996832131609E-16, 0.8070866141732283561 ) ) ;
#41821=CARTESIAN_POINT ( 'NONE',  ( 0.4330708661417322913, 0.1574803149606299191, 1.186023622047243986 ) ) ;
#41827=DIRECTION ( 'NONE',  ( 0.000000000000000000, -1.020425574104001164E-16, 1.000000000000000000 ) ) ;
#41910=CIRCLE ( 'NONE', #14419, 0.1003937007874010356 ) ;
#42011=DIRECTION ( 'NONE',  ( 0.000000000000000000, 0.000000000000000000, -1.000000000000000000 ) ) ;
#42143=CONICAL_SURFACE ( 'NONE', #45213, 0.1003937007874010356, 0.7853981633978559529 ) ;
#42164=AXIS2_PLACEMENT_3D ( 'NONE', #22026, #18426, #10313 ) ;
#42169=FACE_BOUND ( 'NONE', #6882, .T. ) ;
#42303=EDGE_CURVE ( 'NONE', #13605, #4124, #19830, .T. ) ;
#42318=CARTESIAN_POINT ( 'NONE',  ( -0.6195511811023656223, 0.6102362204724407491, 1.186023622047243986 ) ) ;
#42359=LINE ( 'NONE', #23466, #45754 ) ;
#42395=VERTEX_POINT ( 'NONE', #41604 ) ;
#42482=EDGE_LOOP ( 'NONE', ( #35750, #38047, #20470, #2073 ) ) ;
#42535=FACE_BOUND ( 'NONE', #20621, .T. ) ;
#42538=EDGE_CURVE ( 'NONE', #20302, #44293, #29845, .T. ) ;
#42566=VERTEX_POINT ( 'NONE', #15675 ) ;
#42594=DIRECTION ( 'NONE',  ( 0.000000000000000000, 0.000000000000000000, 1.000000000000000000 ) ) ;
#42750=LINE ( 'NONE', #46841, #46753 ) ;
#42784=ORIENTED_EDGE ( 'NONE', *, *, #24727, .T. ) ;
#42823=EDGE_LOOP ( 'NONE', ( #16233, #26997, #30834, #15167 ) ) ;
#42913=VECTOR ( 'NONE', #44409, 39.37007874015748143 ) ;
#42929=ORIENTED_EDGE ( 'NONE', *, *, #35882, .F. ) ;
#42937=DIRECTION ( 'NONE',  ( 0.000000000000000000, 0.000000000000000000, -1.000000000000000000 ) ) ;
#43011=ORIENTED_EDGE ( 'NONE', *, *, #27138, .T. ) ;
#43065=DIRECTION ( 'NONE',  ( -0.000000000000000000, 1.000000000000000000, -0.000000000000000000 ) ) ;
#43084=CIRCLE ( 'NONE', #39256, 0.1968503937007874405 ) ;
#43129=ORIENTED_EDGE ( 'NONE', *, *, #30410, .F. ) ;
#43147=VERTEX_POINT ( 'NONE', #5208 ) ;
#43170=CARTESIAN_POINT ( 'NONE',  ( 0.1377952755905512139, 0.1564960629921262614, 0.7066929133858274037 ) ) ;
#43209=CARTESIAN_POINT ( 'NONE',  ( -0.4330708661417322913, 0.1864803149606299448, 1.186023622047243986 ) ) ;
#43246=DIRECTION ( 'NONE',  ( 1.000000000000000000, 0.000000000000000000, 0.000000000000000000 ) ) ;
#43248=PRODUCT_DEFINITION_SHAPE ( 'NONE', 'NONE',  #11944 ) ;
#43357=VERTEX_POINT ( 'NONE', #29851 ) ;
#43420=DIRECTION ( 'NONE',  ( 0.000000000000000000, 0.000000000000000000, 1.000000000000000000 ) ) ;
#43440=ORIENTED_EDGE ( 'NONE', *, *, #45641, .T. ) ;
#43468=CARTESIAN_POINT ( 'NONE',  ( 0.1377952755905512139, 0.1564960629921262614, 0.7066929133858274037 ) ) ;
#43531=CARTESIAN_POINT ( 'NONE',  ( -0.4620708661417322616, 0.9842519685039375910, -0.7135826771653542844 ) ) ;
#43559=LINE ( 'NONE', #46681, #26814 ) ;
#43603=VECTOR ( 'NONE', #45191, 39.37007874015748143 ) ;
#43655=VERTEX_POINT ( 'NONE', #37462 ) ;
#43669=DIRECTION ( 'NONE',  ( 1.000000000000000000, 0.000000000000000000, 0.000000000000000000 ) ) ;
#43686=EDGE_LOOP ( 'NONE', ( #23079, #9322, #15705, #8709 ) ) ;
#43692=VERTEX_POINT ( 'NONE', #12558 ) ;
#43737=DIRECTION ( 'NONE',  ( -1.000000000000000000, 0.000000000000000000, 0.000000000000000000 ) ) ;
#43806=STYLED_ITEM ( 'NONE', ( #5284 ), #37046 ) ;
#44009=AXIS2_PLACEMENT_3D ( 'NONE', #15298, #44494, #11712 ) ;
#44021=CARTESIAN_POINT ( 'NONE',  ( -0.6195511811023656223, 0.9842519685039370358, -0.7135826771653542844 ) ) ;
#44054=FACE_OUTER_BOUND ( 'NONE', #24082, .T. ) ;
#44163=DIRECTION ( 'NONE',  ( -0.000000000000000000, -0.000000000000000000, -1.000000000000000000 ) ) ;
#44249=VERTEX_POINT ( 'NONE', #22231 ) ;
#44293=VERTEX_POINT ( 'NONE', #14589 ) ;
#44343=DIRECTION ( 'NONE',  ( -0.000000000000000000, 1.000000000000000000, -0.000000000000000000 ) ) ;
#44357=VERTEX_POINT ( 'NONE', #3567 ) ;
#44377=AXIS2_PLACEMENT_3D ( 'NONE', #31857, #46436, #42594 ) ;
#44409=DIRECTION ( 'NONE',  ( 0.000000000000000000, -1.000000000000000000, 0.000000000000000000 ) ) ;
#44494=DIRECTION ( 'NONE',  ( 0.000000000000000000, -0.000000000000000000, -1.000000000000000000 ) ) ;
#44495=EDGE_CURVE ( 'NONE', #42566, #18058, #17242, .T. ) ;
#44501=DIRECTION ( 'NONE',  ( 0.000000000000000000, -1.020425574104001164E-16, 1.000000000000000000 ) ) ;
#44516=CYLINDRICAL_SURFACE ( 'NONE', #22995, 0.1624015748031501782 ) ;
#44562=CONICAL_SURFACE ( 'NONE', #36140, 0.1003937007874010356, 0.7853981633978559529 ) ;
#44647=ORIENTED_EDGE ( 'NONE', *, *, #39860, .T. ) ;
#44775=ORIENTED_EDGE ( 'NONE', *, *, #30651, .T. ) ;
#44808=CARTESIAN_POINT ( 'NONE',  ( 0.1377952755905511861, 0.1574803149606299191, 0.8070866141732283561 ) ) ;
#44859=CARTESIAN_POINT ( 'NONE',  ( 0.1377952755905511861, 0.1564960629921262614, 0.9074803149606294195 ) ) ;
#44870=CARTESIAN_POINT ( 'NONE',  ( 0.4330708661417322913, 0.1574803149606299191, -1.186023622047243986 ) ) ;
#44921=CARTESIAN_POINT ( 'NONE',  ( -0.4620708661417322616, 1.354170115732555191, -0.4197102375732078561 ) ) ;
#44978=DIRECTION ( 'NONE',  ( 0.000000000000000000, 0.000000000000000000, 1.000000000000000000 ) ) ;
#44993=CARTESIAN_POINT ( 'NONE',  ( -0.4330708661417356775, 0.1864803149606299171, 1.186023622047243986 ) ) ;
#45000=ORIENTED_EDGE ( 'NONE', *, *, #25210, .T. ) ;
#45033=CIRCLE ( 'NONE', #21344, 0.1013779527559055538 ) ;
#45182=ORIENTED_EDGE ( 'NONE', *, *, #1123, .T. ) ;
#45191=DIRECTION ( 'NONE',  ( 0.000000000000000000, -1.000000000000000000, 0.000000000000000000 ) ) ;
#45208=CIRCLE ( 'NONE', #42164, 0.1003937007874010356 ) ;
#45213=AXIS2_PLACEMENT_3D ( 'NONE', #14338, #32075, #28983 ) ;
#45277=ORIENTED_EDGE ( 'NONE', *, *, #9307, .F. ) ;
#45315=DIRECTION ( 'NONE',  ( 1.000000000000000000, -0.000000000000000000, -0.000000000000000000 ) ) ;
#45469=DIRECTION ( 'NONE',  ( 1.000000000000000000, 0.000000000000000000, 0.000000000000000000 ) ) ;
#45588=ORIENTED_EDGE ( 'NONE', *, *, #899, .T. ) ;
#45627=EDGE_LOOP ( 'NONE', ( #32827, #18277, #39150, #11510 ) ) ;
#45641=EDGE_CURVE ( 'NONE', #12253, #29994, #30374, .T. ) ;
#45754=VECTOR ( 'NONE', #45469, 39.37007874015748143 ) ;
#45887=CARTESIAN_POINT ( 'NONE',  ( -0.6195511811023656223, 0.1864803149606298893, 1.186023622047243986 ) ) ;
#45904=VECTOR ( 'NONE', #4718, 39.37007874015748143 ) ;
#45910=DIRECTION ( 'NONE',  ( 0.000000000000000000, 1.000000000000000000, 0.000000000000000000 ) ) ;
#46036=VECTOR ( 'NONE', #21845, 39.37007874015748143 ) ;
#46103=DIRECTION ( 'NONE',  ( 0.000000000000000000, 0.000000000000000000, -1.000000000000000000 ) ) ;
#46110=( GEOMETRIC_REPRESENTATION_CONTEXT ( 3 ) GLOBAL_UNCERTAINTY_ASSIGNED_CONTEXT ( ( #29243 ) ) GLOBAL_UNIT_ASSIGNED_CONTEXT ( ( #30026, #29565, #11787 ) ) REPRESENTATION_CONTEXT ( 'NONE', 'WORKASPACE' ) ) ;
#46149=AXIS2_PLACEMENT_3D ( 'NONE', #23894, #45910, #5907 ) ;
#46181=DIRECTION ( 'NONE',  ( 0.000000000000000000, 0.000000000000000000, -1.000000000000000000 ) ) ;
#46223=ORIENTED_EDGE ( 'NONE', *, *, #20772, .T. ) ;
#46224=VERTEX_POINT ( 'NONE', #27177 ) ;
#46225=ORIENTED_EDGE ( 'NONE', *, *, #20513, .F. ) ;
#46399=VERTEX_POINT ( 'NONE', #1732 ) ;
#46436=DIRECTION ( 'NONE',  ( -0.000000000000000000, 1.000000000000000000, -0.000000000000000000 ) ) ;
#46562=EDGE_LOOP ( 'NONE', ( #31926, #32829 ) ) ;
#46577=EDGE_CURVE ( 'NONE', #44293, #529, #18244, .T. ) ;
#46681=CARTESIAN_POINT ( 'NONE',  ( 0.2362204724409448509, 0.1574803149606299191, 1.186023622047243986 ) ) ;
#46753=VECTOR ( 'NONE', #43246, 39.37007874015748143 ) ;
#46828=ADVANCED_FACE ( 'NONE', ( #19362 ), #34645, .F. ) ;
#46841=CARTESIAN_POINT ( 'NONE',  ( -0.6195511811023656223, 0.9842519685039370358, -1.186023622047243986 ) ) ;
#46879=ORIENTED_EDGE ( 'NONE', *, *, #36036, .T. ) ;
#46999=ADVANCED_FACE ( 'NONE', ( #21247 ), #17190, .T. ) ;
#47062=ADVANCED_FACE ( 'NONE', ( #14001 ), #28650, .F. ) ;
#47156=DIRECTION ( 'NONE',  ( 0.000000000000000000, 0.000000000000000000, 1.000000000000000000 ) ) ;
#47161=ORIENTED_EDGE ( 'NONE', *, *, #12634, .T. ) ;
#47167=CIRCLE ( 'NONE', #18079, 0.4724409448818900348 ) ;
#47238=EDGE_CURVE ( 'NONE', #29873, #27278, #12448, .T. ) ;
#47356=ORIENTED_EDGE ( 'NONE', *, *, #1300, .T. ) ;
ENDSEC;
END-ISO-10303-21;
